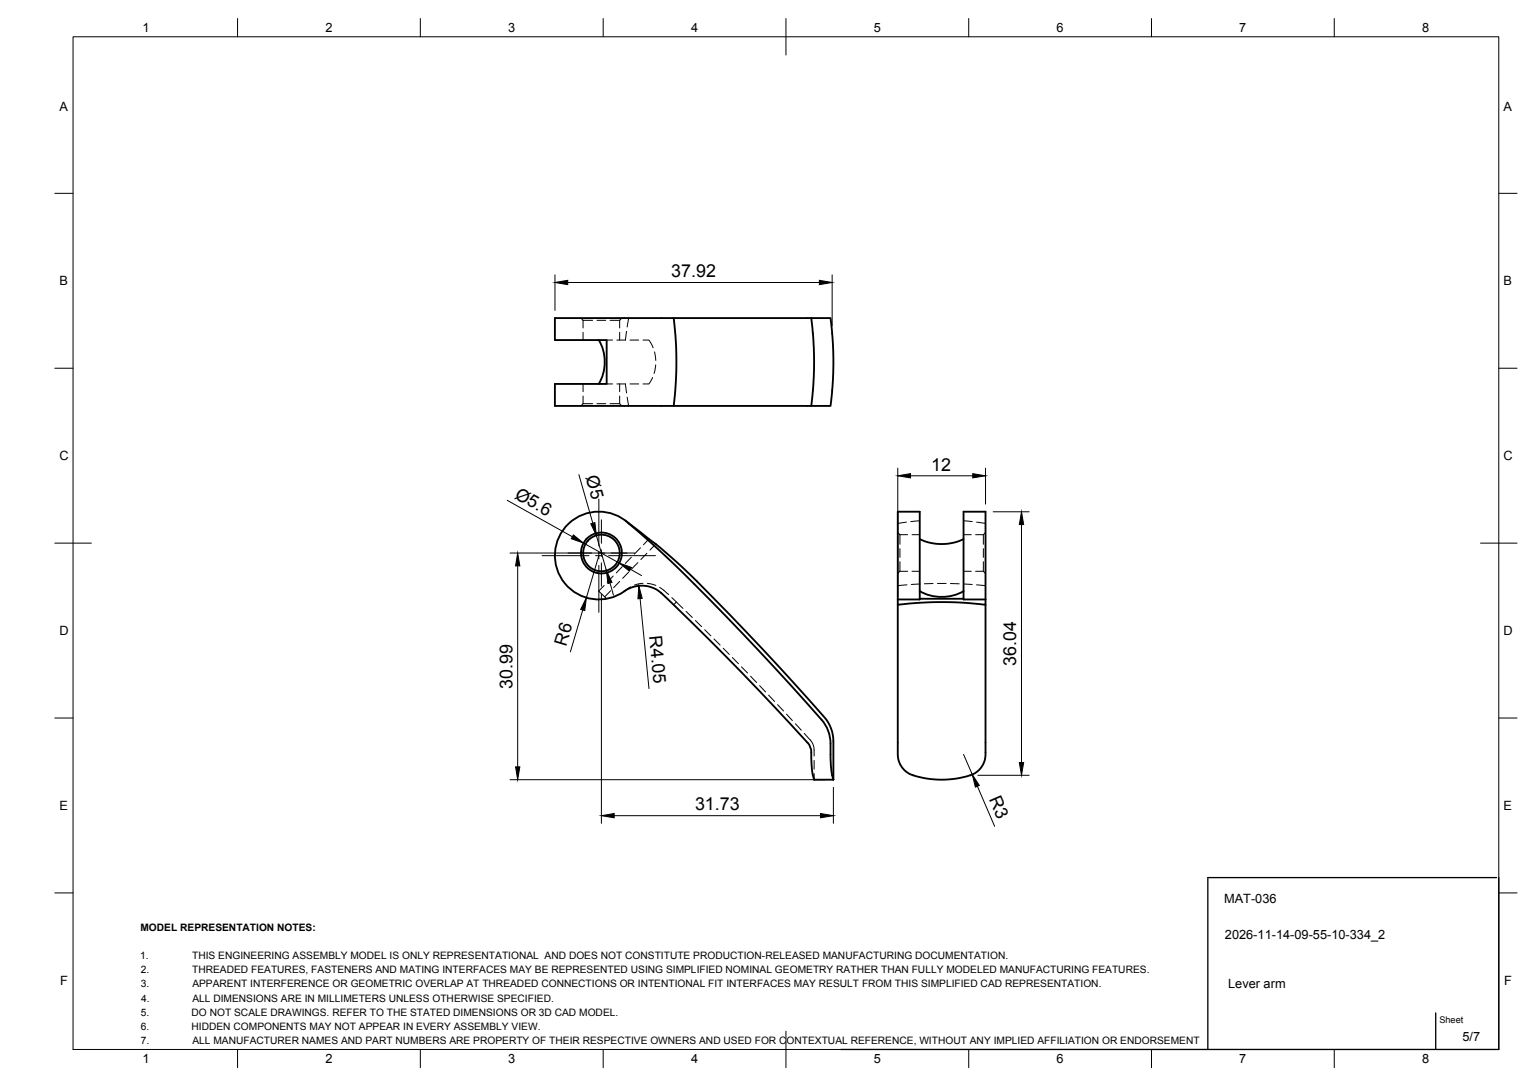
ISO-10303-21;
HEADER;
/* Generated by software containing ST-Developer
 * from STEP Tools, Inc. (www.steptools.com) 
 */

FILE_DESCRIPTION(
/* description */ (''),
/* implementation_level */ '2;1');

FILE_NAME(
/* name */ 'Lever arm.step',
/* time_stamp */ '2026-11-14T09:55:16-08:00',
/* author */ (''),
/* organization */ (''),
/* preprocessor_version */ 'ST-DEVELOPER v20.2',
/* originating_system */ 'Autodesk Translation Framework v15.17.0.0',
/* authorisation */ '');

FILE_SCHEMA (('AUTOMOTIVE_DESIGN { 1 0 10303 214 3 1 1 }'));
ENDSEC;

DATA;
#10=MECHANICAL_DESIGN_GEOMETRIC_PRESENTATION_REPRESENTATION('',(#60),#170250);
#36=B_SPLINE_SURFACE_WITH_KNOTS('',3,3,((#168992,#168993,#168994,#168995),
(#168996,#168997,#168998,#168999),(#169000,#169001,#169002,#169003),(#169004,
#169005,#169006,#169007),(#169008,#169009,#169010,#169011),(#169012,#169013,
#169014,#169015),(#169016,#169017,#169018,#169019),(#169020,#169021,#169022,
#169023),(#169024,#169025,#169026,#169027),(#169028,#169029,#169030,#169031)),
 .UNSPECIFIED.,.F.,.F.,.F.,(4,1,1,1,3,4),(4,4),(0.135790601649557,0.226849968153009,
0.317909334656459,0.40896870115991,0.500028067663362,0.5036704423235),(0.807901539596212,
1.),.UNSPECIFIED.);
#37=B_SPLINE_SURFACE_WITH_KNOTS('',3,3,((#169171,#169172,#169173,#169174,
#169175,#169176,#169177),(#169178,#169179,#169180,#169181,#169182,#169183,
#169184),(#169185,#169186,#169187,#169188,#169189,#169190,#169191),(#169192,
#169193,#169194,#169195,#169196,#169197,#169198),(#169199,#169200,#169201,
#169202,#169203,#169204,#169205),(#169206,#169207,#169208,#169209,#169210,
#169211,#169212),(#169213,#169214,#169215,#169216,#169217,#169218,#169219),
(#169220,#169221,#169222,#169223,#169224,#169225,#169226),(#169227,#169228,
#169229,#169230,#169231,#169232,#169233),(#169234,#169235,#169236,#169237,
#169238,#169239,#169240),(#169241,#169242,#169243,#169244,#169245,#169246,
#169247),(#169248,#169249,#169250,#169251,#169252,#169253,#169254),(#169255,
#169256,#169257,#169258,#169259,#169260,#169261)),.UNSPECIFIED.,.F.,.F.,
 .F.,(4,3,1,1,1,3,4),(4,3,4),(0.114681185572966,0.118496689180301,0.213879533801066,
0.309262378421832,0.404645223042596,0.500028067663362,0.500047049913778),
(-2.58598232202791E-10,0.97179933976621,0.977592668595424),
 .UNSPECIFIED.);
#38=B_SPLINE_SURFACE_WITH_KNOTS('',3,3,((#169612,#169613,#169614,#169615,
#169616,#169617),(#169618,#169619,#169620,#169621,#169622,#169623),(#169624,
#169625,#169626,#169627,#169628,#169629),(#169630,#169631,#169632,#169633,
#169634,#169635),(#169636,#169637,#169638,#169639,#169640,#169641),(#169642,
#169643,#169644,#169645,#169646,#169647),(#169648,#169649,#169650,#169651,
#169652,#169653),(#169654,#169655,#169656,#169657,#169658,#169659),(#169660,
#169661,#169662,#169663,#169664,#169665),(#169666,#169667,#169668,#169669,
#169670,#169671),(#169672,#169673,#169674,#169675,#169676,#169677),(#169678,
#169679,#169680,#169681,#169682,#169683)),.UNSPECIFIED.,.F.,.F.,.F.,(4,
1,1,1,2,1,1,1,4),(4,2,4),(0.618524756843663,0.666209162238205,0.713893567632747,
0.761577973027289,0.809262378421831,0.856946783816374,0.904631189210916,
0.952315594605458,1.),(0.,0.931730586032522,0.937129966266598),
 .UNSPECIFIED.);
#39=B_SPLINE_SURFACE_WITH_KNOTS('',3,3,((#169891,#169892,#169893,#169894),
(#169895,#169896,#169897,#169898),(#169899,#169900,#169901,#169902),(#169903,
#169904,#169905,#169906),(#169907,#169908,#169909,#169910),(#169911,#169912,
#169913,#169914),(#169915,#169916,#169917,#169918),(#169919,#169920,#169921,
#169922),(#169923,#169924,#169925,#169926),(#169927,#169928,#169929,#169930),
(#169931,#169932,#169933,#169934),(#169935,#169936,#169937,#169938),(#169939,
#169940,#169941,#169942),(#169943,#169944,#169945,#169946),(#169947,#169948,
#169949,#169950)),.UNSPECIFIED.,.F.,.F.,.F.,(4,3,1,1,1,2,1,1,1,4),(4,4),
(0.632176856006048,0.635818669312919,0.681341335648804,0.726864001984689,
0.772386668320574,0.81790933465646,0.863432000992345,0.90895466732823,0.954477333664115,
1.),(0.0153819466590792,1.),.UNSPECIFIED.);
#46=SHAPE_REPRESENTATION_RELATIONSHIP('SRR','None',#170278,#52);
#52=ADVANCED_BREP_SHAPE_REPRESENTATION('',(#66),#170246);
#60=STYLED_ITEM('',(#170316),#66);
#66=MANIFOLD_SOLID_BREP('Body1',#71400);
#76=FACE_BOUND('',#15893,.T.);
#77=FACE_BOUND('',#15895,.T.);
#78=FACE_BOUND('',#15897,.T.);
#79=FACE_BOUND('',#15901,.T.);
#98=PLANE('',#77702);
#99=PLANE('',#77704);
#100=PLANE('',#77706);
#101=PLANE('',#77707);
#102=PLANE('',#77710);
#192=ELLIPSE('',#77705,65.55169862647,42.389902647677);
#193=ELLIPSE('',#77708,65.5506952259048,42.388915448489);
#4370=(
BOUNDED_SURFACE()
B_SPLINE_SURFACE(3,1,((#168511,#168512),(#168513,#168514),(#168515,#168516),
(#168517,#168518)),.UNSPECIFIED.,.F.,.F.,.F.)
B_SPLINE_SURFACE_WITH_KNOTS((4,4),(2,2),(-8.56707287333166E-8,1.00000008548767),
(0.00592879452423504,0.99406998347921),.UNSPECIFIED.)
GEOMETRIC_REPRESENTATION_ITEM()
RATIONAL_B_SPLINE_SURFACE(((1.00000000253644,1.00000000253644),(0.990131033425531,
0.990131033425531),(0.990131033423724,0.990131033423724),(1.00000000253103,
1.00000000253102)))
REPRESENTATION_ITEM('')
SURFACE()
);
#4371=(
BOUNDED_SURFACE()
B_SPLINE_SURFACE(3,2,((#168680,#168681,#168682),(#168683,#168684,#168685),
(#168686,#168687,#168688),(#168689,#168690,#168691),(#168692,#168693,#168694),
(#168695,#168696,#168697),(#168698,#168699,#168700),(#168701,#168702,#168703),
(#168704,#168705,#168706),(#168707,#168708,#168709),(#168710,#168711,#168712),
(#168713,#168714,#168715),(#168716,#168717,#168718),(#168719,#168720,#168721),
(#168722,#168723,#168724),(#168725,#168726,#168727),(#168728,#168729,#168730),
(#168731,#168732,#168733),(#168734,#168735,#168736),(#168737,#168738,#168739),
(#168740,#168741,#168742),(#168743,#168744,#168745),(#168746,#168747,#168748),
(#168749,#168750,#168751),(#168752,#168753,#168754),(#168755,#168756,#168757),
(#168758,#168759,#168760),(#168761,#168762,#168763),(#168764,#168765,#168766),
(#168767,#168768,#168769),(#168770,#168771,#168772),(#168773,#168774,#168775),
(#168776,#168777,#168778),(#168779,#168780,#168781),(#168782,#168783,#168784),
(#168785,#168786,#168787),(#168788,#168789,#168790),(#168791,#168792,#168793),
(#168794,#168795,#168796),(#168797,#168798,#168799),(#168800,#168801,#168802),
(#168803,#168804,#168805),(#168806,#168807,#168808),(#168809,#168810,#168811),
(#168812,#168813,#168814),(#168815,#168816,#168817),(#168818,#168819,#168820),
(#168821,#168822,#168823),(#168824,#168825,#168826),(#168827,#168828,#168829)),
 .UNSPECIFIED.,.F.,.F.,.F.)
B_SPLINE_SURFACE_WITH_KNOTS((4,2,2,2,2,2,2,2,2,2,2,2,2,2,2,2,2,2,2,2,2,
2,2,2,4),(3,3),(0.00438204809785496,0.00442773757395586,0.00445058231200631,
0.00446200468103154,0.00447342705005676,0.00451911652615766,0.00454196126420811,
0.00456480600225856,0.00474756390666215,0.00511307971546933,0.0058441113330837,
0.00730617456831243,0.0102303010387699,0.0131544275092274,0.0146164907444561,
0.0153475223620705,0.0157130381708776,0.0158957960752812,0.0159186408133317,
0.0159414855513821,0.015987175027483,0.0159985973965083,0.0160100197655335,
0.0160328645035839,0.0160785539796848),(0.,1.),.UNSPECIFIED.)
GEOMETRIC_REPRESENTATION_ITEM()
RATIONAL_B_SPLINE_SURFACE(((1.,0.934218767962417,1.),(1.,0.934219268725543,
1.),(1.,0.934219769475696,1.),(1.,0.934220520581468,1.),(1.,0.934221098516136,
1.),(1.,0.93422098270531,1.),(1.,0.934218146084782,1.),(1.,0.934214890227589,
1.),(1.,0.934213259806577,1.),(1.,0.934205095242336,1.),(1.,0.934198523721367,
1.),(1.,0.934188606688787,1.),(1.,0.934185286091514,1.),(1.,0.934178648365384,
1.),(1.,0.934175336166584,1.),(1.,0.934145586350039,1.),(1.,0.934119568538277,
1.),(1.,0.934042793646304,1.),(1.,0.933993312945644,1.),(1.,0.933849992791617,
1.),(1.,0.933761355730532,1.),(1.,0.93351603018512,1.),(1.,0.933379914807182,
1.),(1.,0.93305317905279,1.),(1.,0.932943966614937,1.),(1.,0.932943963043387,
1.),(1.,0.933053175643618,1.),(1.,0.933379911515294,1.),(1.,0.93351602735766,
1.),(1.,0.933761354538682,1.),(1.,0.933849992301547,1.),(1.,0.933993313783528,
1.),(1.,0.93404279394322,1.),(1.,0.934119568707732,1.),(1.,0.934145586476303,
1.),(1.,0.934175336243606,1.),(1.,0.934178648436936,1.),(1.,0.934185286152106,
1.),(1.,0.934188606743602,1.),(1.,0.934198523759289,1.),(1.,0.9342050952691,
1.),(1.,0.934213259819631,1.),(1.,0.934214890237893,1.),(1.,0.934218146089636,
1.),(1.,0.934220982704232,1.),(1.,0.934221098518431,1.),(1.,0.934220520582345,
1.),(1.,0.934219769477844,1.),(1.,0.934219268728507,1.),(1.,0.934218767966226,
1.)))
REPRESENTATION_ITEM('')
SURFACE()
);
#4372=(
BOUNDED_SURFACE()
B_SPLINE_SURFACE(3,1,((#168914,#168915),(#168916,#168917),(#168918,#168919),
(#168920,#168921)),.UNSPECIFIED.,.F.,.F.,.F.)
B_SPLINE_SURFACE_WITH_KNOTS((4,4),(2,2),(-8.59560614834357E-8,1.00000008613876),
(0.00592875831867496,0.994072405691805),.UNSPECIFIED.)
GEOMETRIC_REPRESENTATION_ITEM()
RATIONAL_B_SPLINE_SURFACE(((1.00000000254489,1.00000000254489),(0.990131033419105,
0.990131033419106),(0.990131033420908,0.990131033420909),(1.0000000025503,
1.0000000025503)))
REPRESENTATION_ITEM('')
SURFACE()
);
#4373=(
BOUNDED_SURFACE()
B_SPLINE_SURFACE(3,2,((#169270,#169271,#169272),(#169273,#169274,#169275),
(#169276,#169277,#169278),(#169279,#169280,#169281),(#169282,#169283,#169284),
(#169285,#169286,#169287),(#169288,#169289,#169290),(#169291,#169292,#169293),
(#169294,#169295,#169296),(#169297,#169298,#169299),(#169300,#169301,#169302),
(#169303,#169304,#169305),(#169306,#169307,#169308),(#169309,#169310,#169311),
(#169312,#169313,#169314),(#169315,#169316,#169317),(#169318,#169319,#169320),
(#169321,#169322,#169323),(#169324,#169325,#169326),(#169327,#169328,#169329),
(#169330,#169331,#169332),(#169333,#169334,#169335),(#169336,#169337,#169338),
(#169339,#169340,#169341),(#169342,#169343,#169344),(#169345,#169346,#169347),
(#169348,#169349,#169350),(#169351,#169352,#169353),(#169354,#169355,#169356),
(#169357,#169358,#169359),(#169360,#169361,#169362),(#169363,#169364,#169365),
(#169366,#169367,#169368),(#169369,#169370,#169371),(#169372,#169373,#169374),
(#169375,#169376,#169377),(#169378,#169379,#169380),(#169381,#169382,#169383),
(#169384,#169385,#169386),(#169387,#169388,#169389),(#169390,#169391,#169392),
(#169393,#169394,#169395),(#169396,#169397,#169398),(#169399,#169400,#169401),
(#169402,#169403,#169404),(#169405,#169406,#169407),(#169408,#169409,#169410),
(#169411,#169412,#169413),(#169414,#169415,#169416),(#169417,#169418,#169419),
(#169420,#169421,#169422),(#169423,#169424,#169425),(#169426,#169427,#169428),
(#169429,#169430,#169431),(#169432,#169433,#169434),(#169435,#169436,#169437),
(#169438,#169439,#169440),(#169441,#169442,#169443),(#169444,#169445,#169446),
(#169447,#169448,#169449),(#169450,#169451,#169452),(#169453,#169454,#169455),
(#169456,#169457,#169458),(#169459,#169460,#169461),(#169462,#169463,#169464),
(#169465,#169466,#169467),(#169468,#169469,#169470),(#169471,#169472,#169473),
(#169474,#169475,#169476),(#169477,#169478,#169479),(#169480,#169481,#169482),
(#169483,#169484,#169485),(#169486,#169487,#169488),(#169489,#169490,#169491)),
 .UNSPECIFIED.,.F.,.F.,.F.)
B_SPLINE_SURFACE_WITH_KNOTS((4,2,2,2,2,2,2,2,2,2,2,2,2,2,2,2,2,2,2,2,2,
2,2,2,2,2,2,2,2,2,2,2,2,2,2,2,4),(3,3),(0.0179612750605611,0.0180038120055911,
0.0180250804781061,0.0180303975962348,0.0180357147143635,0.018046348950621,
0.0181314228406809,0.0182164967307408,0.0182271309669983,0.0182377652032558,
0.0182590336757708,0.0183015706208007,0.0186418661810403,0.0193224573015194,
0.0200030484219985,0.0206836395424776,0.0213642306629567,0.0220448217834359,
0.0234060040243941,0.0247671862653523,0.0254477773858315,0.0261283685063106,
0.0268089596267897,0.0274895507472688,0.0281701418677479,0.0285104374279875,
0.0285529743730174,0.0285742428455324,0.0285848770817899,0.0285955113180474,
0.0286805852081073,0.0287656590981672,0.0287762933344247,0.0287816104525534,
0.0287869275706821,0.0288081960431971,0.0288507329882271),(0.,1.),
 .UNSPECIFIED.)
GEOMETRIC_REPRESENTATION_ITEM()
RATIONAL_B_SPLINE_SURFACE(((1.,0.936904821453696,1.),(1.,0.936904794108661,
1.),(1.,0.936904766764048,1.),(1.,0.936904725747745,1.),(1.,0.936905128260374,
1.),(1.,0.936904590939729,1.),(1.,0.936903346459592,1.),(1.,0.936901627765994,
1.),(1.,0.936900767797278,1.),(1.,0.936898186025644,1.),(1.,0.936896462357224,
1.),(1.,0.936880926961442,1.),(1.,0.936866958574279,1.),(1.,0.936838704163249,
1.),(1.,0.936824418139244,1.),(1.,0.936808168049907,1.),(1.,0.936806360007847,
1.),(1.,0.936802738971814,1.),(1.,0.936800862095946,1.),(1.,0.936795849431034,
1.),(1.,0.936792514575336,1.),(1.,0.936782530740213,1.),(1.,0.936775902492467,
1.),(1.,0.936716496356665,1.),(1.,0.936665452813206,1.),(1.,0.936517538966925,
1.),(1.,0.93642586040289,1.),(1.,0.936256634386565,1.),(1.,0.936179189842934,
1.),(1.,0.936038226722045,1.),(1.,0.935974776717855,1.),(1.,0.935862123528188,
1.),(1.,0.935812981619732,1.),(1.,0.93572859095576,1.),(1.,0.935693341074582,
1.),(1.,0.935608906032864,1.),(1.,0.935580787501173,1.),(1.,0.935580755598083,
1.),(1.,0.935608926183175,1.),(1.,0.935693493416876,1.),(1.,0.935728787043659,
1.),(1.,0.935813225027166,1.),(1.,0.935862370889367,1.),(1.,0.935974951078453,
1.),(1.,0.936038323852223,1.),(1.,0.936179015169328,1.),(1.,0.93625634937854,
1.),(1.,0.936425491452454,1.),(1.,0.936517220625567,1.),(1.,0.936665263045723,
1.),(1.,0.9367163495052,1.),(1.,0.936775803162665,1.),(1.,0.936782436680194,
1.),(1.,0.936792428402367,1.),(1.,0.936795765884152,1.),(1.,0.936800782483542,
1.),(1.,0.936802654166495,1.),(1.,0.936806278312161,1.),(1.,0.936808087904325,
1.),(1.,0.936824351902175,1.),(1.,0.936838649987733,1.),(1.,0.936866927922814,
1.),(1.,0.936880907772467,1.),(1.,0.93689645572885,1.),(1.,0.936898180788246,
1.),(1.,0.936900764639372,1.),(1.,0.936901625300091,1.),(1.,0.936903345375374,
1.),(1.,0.936904591114425,1.),(1.,0.936905127567446,1.),(1.,0.936904725770864,
1.),(1.,0.936904766820085,1.),(1.,0.93690479418665,1.),(1.,0.936904821553629,
1.)))
REPRESENTATION_ITEM('')
SURFACE()
);
#4374=(
BOUNDED_SURFACE()
B_SPLINE_SURFACE(3,2,((#169695,#169696,#169697),(#169698,#169699,#169700),
(#169701,#169702,#169703),(#169704,#169705,#169706),(#169707,#169708,#169709),
(#169710,#169711,#169712),(#169713,#169714,#169715),(#169716,#169717,#169718),
(#169719,#169720,#169721),(#169722,#169723,#169724),(#169725,#169726,#169727),
(#169728,#169729,#169730),(#169731,#169732,#169733),(#169734,#169735,#169736),
(#169737,#169738,#169739),(#169740,#169741,#169742),(#169743,#169744,#169745),
(#169746,#169747,#169748),(#169749,#169750,#169751),(#169752,#169753,#169754),
(#169755,#169756,#169757),(#169758,#169759,#169760),(#169761,#169762,#169763),
(#169764,#169765,#169766),(#169767,#169768,#169769),(#169770,#169771,#169772),
(#169773,#169774,#169775),(#169776,#169777,#169778),(#169779,#169780,#169781),
(#169782,#169783,#169784),(#169785,#169786,#169787),(#169788,#169789,#169790),
(#169791,#169792,#169793),(#169794,#169795,#169796),(#169797,#169798,#169799),
(#169800,#169801,#169802),(#169803,#169804,#169805),(#169806,#169807,#169808),
(#169809,#169810,#169811),(#169812,#169813,#169814),(#169815,#169816,#169817),
(#169818,#169819,#169820),(#169821,#169822,#169823),(#169824,#169825,#169826),
(#169827,#169828,#169829),(#169830,#169831,#169832),(#169833,#169834,#169835),
(#169836,#169837,#169838),(#169839,#169840,#169841),(#169842,#169843,#169844),
(#169845,#169846,#169847),(#169848,#169849,#169850)),.UNSPECIFIED.,.F.,
 .F.,.F.)
B_SPLINE_SURFACE_WITH_KNOTS((4,2,2,2,2,2,2,2,2,2,2,2,2,2,2,2,2,2,2,2,2,
2,2,2,2,4),(3,3),(0.0156015153159842,0.0159832133339201,0.0161740623428881,
0.016269486847372,0.016317199099614,0.016341055225735,0.0163529832887955,
0.016364911351856,0.0171283073877279,0.0186550994594716,0.0194184954953434,
0.0201818915312153,0.021708683602959,0.0224720796388308,0.0232354756747027,
0.0247622677464464,0.0262890598181901,0.0270524558540619,0.0270584198855922,
0.0270643839171224,0.0270763119801829,0.0271001681063039,0.0271478803585459,
0.0272433048630299,0.0274341538719979,0.0278158518899338),(0.,1.),
 .UNSPECIFIED.)
GEOMETRIC_REPRESENTATION_ITEM()
RATIONAL_B_SPLINE_SURFACE(((1.,0.776444097652961,1.),(1.,0.776058926606058,
1.),(1.,0.775673843099958,1.),(1.,0.775096481210286,1.),(1.,0.774904071156476,
1.),(1.,0.774615538680226,1.),(1.,0.774519374957158,1.),(1.,0.774375152135543,
1.),(1.,0.774327081655569,1.),(1.,0.774254981891155,1.),(1.,0.774230949628936,
1.),(1.,0.774194902757698,1.),(1.,0.774182887387605,1.),(1.,0.774158857160334,
1.),(1.,0.774150992177244,1.),(1.,0.773543654478887,1.),(1.,0.77298505575604,
1.),(1.,0.771431978714256,1.),(1.,0.77056039765908,1.),(1.,0.769511352915782,
1.),(1.,0.769204886519117,1.),(1.,0.768679727581747,1.),(1.,0.768460849050857,
1.),(1.,0.767935355999606,1.),(1.,0.767759786976898,1.),(1.,0.767759465570472,
1.),(1.,0.767803217713065,1.),(1.,0.767978602526777,1.),(1.,0.768110252004706,
1.),(1.,0.768636034778269,1.),(1.,0.769161202927011,1.),(1.,0.770557236848331,
1.),(1.,0.771427908462379,1.),(1.,0.772982352753207,1.),(1.,0.773541690771539,
1.),(1.,0.774144848886315,1.),(1.,0.774149526925736,1.),(1.,0.774158887792997,
1.),(1.,0.77416299521755,1.),(1.,0.774181034357718,1.),(1.,0.774193060706593,
1.),(1.,0.774229140511077,1.),(1.,0.774253194724663,1.),(1.,0.774325360330513,
1.),(1.,0.774373474688076,1.),(1.,0.774517829090711,1.),(1.,0.774614080465712,
1.),(1.,0.774902875681382,1.),(1.,0.775095460606343,1.),(1.,0.775673346165181,
1.),(1.,0.776058777525586,1.),(1.,0.776444294966368,1.)))
REPRESENTATION_ITEM('')
SURFACE()
);
#4458=(
BOUNDED_CURVE()
B_SPLINE_CURVE(3,(#168924,#168925,#168926,#168927,#168928,#168929,#168930,
#168931,#168932,#168933,#168934,#168935,#168936,#168937,#168938,#168939,
#168940,#168941,#168942,#168943,#168944,#168945,#168946,#168947,#168948,
#168949,#168950,#168951,#168952,#168953,#168954,#168955,#168956,#168957,
#168958,#168959,#168960,#168961,#168962,#168963,#168964,#168965,#168966,
#168967,#168968,#168969,#168970,#168971,#168972,#168973,#168974,#168975,
#168976,#168977,#168978,#168979,#168980,#168981,#168982,#168983,#168984,
#168985,#168986,#168987,#168988,#168989),.UNSPECIFIED.,.F.,.F.)
B_SPLINE_CURVE_WITH_KNOTS((4,2,2,2,2,2,2,2,2,2,2,2,2,2,2,2,2,2,2,2,2,2,
2,2,2,2,2,2,2,2,2,2,4),(0.,0.000426248299516627,0.000920386532912638,0.00190866299971401,
0.00981487473411692,0.0177210864685195,0.0187093629353212,0.0196976394021223,
0.0216741923357257,0.0256272982029221,0.0572521451405331,0.120501839015745,
0.183751532890957,0.24700122676617,0.310250920641382,0.373500614516604,
0.500000002267029,0.626499390017453,0.689749083892675,0.752998777767887,
0.816248471643099,0.879498165518312,0.942747859393524,0.974372706331135,
0.978325812198331,0.980302365131934,0.981290641598736,0.982278918065537,
0.99018512979994,0.998091341534343,0.999079618001144,0.99957375623454,1.),
 .UNSPECIFIED.)
CURVE()
GEOMETRIC_REPRESENTATION_ITEM()
RATIONAL_B_SPLINE_CURVE((0.999999893495044,0.999999893494474,0.999999893492739,
0.999999893490038,0.999999893488586,0.999999893484228,0.999999893481318,
0.999999893455095,0.999999893431516,0.999999893383822,0.999999893359708,
0.999999893332278,0.999999893329226,0.999999893323113,0.999999893319945,
0.999999893311484,0.999999893305855,0.999999893289002,0.999999893277814,
0.999999893177536,0.999999893091374,0.999999892841696,0.999999892686943,
0.99999989240129,0.999999892270563,0.999999892032618,0.999999891925514,
0.999999891735356,0.999999891652404,0.999999891509953,0.999999891450451,
0.999999891307925,0.999999891260461,0.999999891260407,0.999999891307959,
0.999999891450708,0.999999891510284,0.999999891652815,0.999999891735774,
0.999999891925809,0.999999892032782,0.999999892270268,0.999999892400809,
0.99999989268632,0.999999892841159,0.999999893091054,0.999999893177288,
0.999999893277646,0.999999893288843,0.999999893305709,0.999999893311343,
0.999999893319811,0.99999989332297,0.999999893329088,0.999999893332142,
0.999999893359596,0.999999893383731,0.999999893431464,0.999999893455062,
0.999999893481307,0.999999893484219,0.99999989348858,0.999999893490033,
0.999999893492737,0.999999893494474,0.999999893495044))
REPRESENTATION_ITEM('')
);
#5369=CYLINDRICAL_SURFACE('',#77682,2.5);
#5370=CYLINDRICAL_SURFACE('',#77689,2.5);
#5371=CYLINDRICAL_SURFACE('',#77691,12.9999999996215);
#5372=CYLINDRICAL_SURFACE('',#77694,6.00000000044796);
#5373=CYLINDRICAL_SURFACE('',#77699,2.99999999919632);
#5374=CYLINDRICAL_SURFACE('',#77700,2.99999999919632);
#5375=CYLINDRICAL_SURFACE('',#77709,4.50000000012307);
#10604=FACE_OUTER_BOUND('',#15875,.T.);
#10605=FACE_OUTER_BOUND('',#15876,.T.);
#10606=FACE_OUTER_BOUND('',#15877,.T.);
#10607=FACE_OUTER_BOUND('',#15878,.T.);
#10608=FACE_OUTER_BOUND('',#15879,.T.);
#10609=FACE_OUTER_BOUND('',#15880,.T.);
#10610=FACE_OUTER_BOUND('',#15881,.T.);
#10611=FACE_OUTER_BOUND('',#15882,.T.);
#10612=FACE_OUTER_BOUND('',#15883,.T.);
#10613=FACE_OUTER_BOUND('',#15884,.T.);
#10614=FACE_OUTER_BOUND('',#15885,.T.);
#10615=FACE_OUTER_BOUND('',#15886,.T.);
#10616=FACE_OUTER_BOUND('',#15887,.T.);
#10617=FACE_OUTER_BOUND('',#15888,.T.);
#10618=FACE_OUTER_BOUND('',#15889,.T.);
#10619=FACE_OUTER_BOUND('',#15890,.T.);
#10620=FACE_OUTER_BOUND('',#15891,.T.);
#10621=FACE_OUTER_BOUND('',#15892,.T.);
#10622=FACE_OUTER_BOUND('',#15894,.T.);
#10623=FACE_OUTER_BOUND('',#15896,.T.);
#10624=FACE_OUTER_BOUND('',#15898,.T.);
#10625=FACE_OUTER_BOUND('',#15899,.T.);
#10626=FACE_OUTER_BOUND('',#15900,.T.);
#15875=EDGE_LOOP('',(#65778,#65779,#65780,#65781,#65782));
#15876=EDGE_LOOP('',(#65783,#65784,#65785,#65786));
#15877=EDGE_LOOP('',(#65787,#65788,#65789,#65790));
#15878=EDGE_LOOP('',(#65791,#65792,#65793,#65794));
#15879=EDGE_LOOP('',(#65795,#65796,#65797,#65798,#65799));
#15880=EDGE_LOOP('',(#65800,#65801,#65802,#65803,#65804,#65805,#65806,#65807));
#15881=EDGE_LOOP('',(#65808,#65809,#65810,#65811,#65812,#65813));
#15882=EDGE_LOOP('',(#65814,#65815,#65816,#65817));
#15883=EDGE_LOOP('',(#65818,#65819,#65820,#65821));
#15884=EDGE_LOOP('',(#65822,#65823,#65824,#65825));
#15885=EDGE_LOOP('',(#65826,#65827,#65828,#65829,#65830,#65831));
#15886=EDGE_LOOP('',(#65832,#65833,#65834,#65835));
#15887=EDGE_LOOP('',(#65836,#65837,#65838,#65839));
#15888=EDGE_LOOP('',(#65840,#65841,#65842,#65843));
#15889=EDGE_LOOP('',(#65844,#65845,#65846,#65847));
#15890=EDGE_LOOP('',(#65848,#65849,#65850,#65851));
#15891=EDGE_LOOP('',(#65852,#65853,#65854,#65855));
#15892=EDGE_LOOP('',(#65856,#65857,#65858,#65859));
#15893=EDGE_LOOP('',(#65860));
#15894=EDGE_LOOP('',(#65861,#65862,#65863,#65864,#65865,#65866,#65867,#65868,
#65869,#65870,#65871));
#15895=EDGE_LOOP('',(#65872));
#15896=EDGE_LOOP('',(#65873,#65874,#65875,#65876,#65877,#65878,#65879,#65880,
#65881,#65882,#65883));
#15897=EDGE_LOOP('',(#65884));
#15898=EDGE_LOOP('',(#65885,#65886,#65887,#65888,#65889,#65890,#65891,#65892));
#15899=EDGE_LOOP('',(#65893,#65894,#65895,#65896));
#15900=EDGE_LOOP('',(#65897,#65898,#65899,#65900));
#15901=EDGE_LOOP('',(#65901));
#21011=CIRCLE('',#77683,2.5);
#21012=CIRCLE('',#77684,2.5);
#21013=CIRCLE('',#77685,2.5);
#21014=CIRCLE('',#77687,2.50000000008162);
#21015=CIRCLE('',#77688,2.79999999966249);
#21016=CIRCLE('',#77690,2.5);
#21017=CIRCLE('',#77693,2.79999999971483);
#21018=CIRCLE('',#77695,6.00000000044796);
#21019=CIRCLE('',#77696,6.00000000044796);
#21020=CIRCLE('',#77697,6.00000000044794);
#21021=CIRCLE('',#77698,6.00000000044795);
#21022=CIRCLE('',#77701,35.000000093214);
#21023=CIRCLE('',#77703,4.50000000012307);
#24318=B_SPLINE_CURVE_WITH_KNOTS('',3,(#168405,#168406,#168407,#168408,
#168409,#168410,#168411,#168412,#168413,#168414),.UNSPECIFIED.,.F.,.F.,
(4,2,2,2,4),(9.99999999599415E-7,0.199896964270254,0.396819956928882,0.593738515946119,
0.793630665235622),.UNSPECIFIED.);
#24319=B_SPLINE_CURVE_WITH_KNOTS('',3,(#168418,#168419,#168420,#168421,
#168422,#168423,#168424,#168425,#168426,#168427),.UNSPECIFIED.,.F.,.F.,
(4,2,2,2,4),(1.0000000102557E-6,0.212494298875736,0.396821009247289,0.581148812864389,
0.793634316910742),.UNSPECIFIED.);
#24320=B_SPLINE_CURVE_WITH_KNOTS('',3,(#168438,#168439,#168440,#168441,
#168442,#168443),.UNSPECIFIED.,.F.,.F.,(4,2,4),(3.14399518292747E-10,0.174984677416615,
0.304359067388048),.UNSPECIFIED.);
#24321=B_SPLINE_CURVE_WITH_KNOTS('',3,(#168451,#168452,#168453,#168454,
#168455,#168456),.UNSPECIFIED.,.F.,.F.,(4,2,4),(0.000105555394099198,0.130107181442079,
0.280405013941638),.UNSPECIFIED.);
#24322=B_SPLINE_CURVE_WITH_KNOTS('',3,(#168459,#168460,#168461,#168462,
#168463,#168464,#168465,#168466,#168467,#168468,#168469,#168470,#168471,
#168472,#168473,#168474,#168475,#168476,#168477,#168478,#168479,#168480,
#168481,#168482,#168483,#168484,#168485,#168486,#168487,#168488,#168489,
#168490,#168491,#168492,#168493,#168494,#168495,#168496,#168497,#168498,
#168499,#168500,#168501,#168502,#168503,#168504,#168505,#168506,#168507,
#168508,#168509,#168510),.UNSPECIFIED.,.F.,.F.,(4,2,2,2,2,2,2,2,2,2,2,2,
2,2,2,2,2,2,2,2,2,2,2,2,2,4),(0.,0.0256250094143976,0.0414375088162371,
0.0493437585171568,0.053296883367617,0.0552734457928468,0.0562617270054617,
0.056755867611765,0.0572500082180766,0.120500005825418,0.247000001040109,
0.373499996254801,0.43674999386215,0.499999991469491,0.626499986684183,
0.689749984291532,0.752999981898873,0.879499977113565,0.942749974720914,
0.943738255933529,0.944726537146144,0.946703099571374,0.950656224421834,
0.958562474122746,0.974374973524585,0.999999995455179),.UNSPECIFIED.);
#24323=B_SPLINE_CURVE_WITH_KNOTS('',3,(#168520,#168521,#168522,#168523,
#168524,#168525,#168526,#168527,#168528,#168529),.UNSPECIFIED.,.F.,.F.,
(4,2,2,2,4),(-0.381457606174089,-0.304035109378442,-0.190979808271481,-0.0912225470703838,
-1.00000006925116E-6),.UNSPECIFIED.);
#24324=B_SPLINE_CURVE_WITH_KNOTS('',3,(#168533,#168534,#168535,#168536,
#168537,#168538,#168539,#168540,#168541,#168542,#168543,#168544,#168545,
#168546,#168547,#168548,#168549,#168550,#168551,#168552,#168553,#168554,
#168555,#168556,#168557,#168558,#168559,#168560,#168561,#168562,#168563,
#168564,#168565,#168566,#168567,#168568,#168569,#168570,#168571,#168572,
#168573,#168574,#168575,#168576,#168577,#168578,#168579,#168580,#168581,
#168582,#168583,#168584,#168585,#168586,#168587,#168588,#168589,#168590,
#168591,#168592,#168593,#168594,#168595,#168596,#168597,#168598,#168599,
#168600,#168601,#168602,#168603,#168604,#168605,#168606,#168607,#168608,
#168609,#168610,#168611,#168612,#168613,#168614,#168615,#168616,#168617,
#168618,#168619,#168620,#168621,#168622,#168623,#168624,#168625,#168626,
#168627,#168628,#168629,#168630,#168631,#168632,#168633,#168634,#168635,
#168636,#168637,#168638,#168639,#168640,#168641),.UNSPECIFIED.,.F.,.F.,
(4,3,3,3,3,3,3,3,3,3,3,3,3,3,3,3,3,3,3,3,3,3,3,3,3,3,3,3,3,3,3,3,3,3,3,
3,4),(0.,0.000877428960298162,0.00182186904808312,0.00560425316389786,0.00749819548399555,
0.00939395278983934,0.0246236265420485,0.0553976406888011,0.10510590613333,
0.117953721761098,0.16822163443711,0.218581997077039,0.244710640454446,
0.25,0.350381617416015,0.448693290958287,0.484375,0.498632474707576,0.49999999286025,
0.50105084551746,0.601647811048279,0.624999999999999,0.725405038227879,
0.746093749999999,0.749999999999999,0.753208507973121,0.875,0.883895257725269,
0.918382175878415,0.946288347314178,0.976389806038248,0.991048440539466,
0.99286064175195,0.994668244628355,0.998269520917499,0.999166914580596,
0.999999987137999),.UNSPECIFIED.);
#24325=B_SPLINE_CURVE_WITH_KNOTS('',3,(#168644,#168645,#168646,#168647,
#168648,#168649,#168650,#168651,#168652,#168653),.UNSPECIFIED.,.F.,.F.,
(4,2,2,2,4),(-0.381485937812174,-0.290460031477783,-0.190961318136168,-0.0775891327103021,
-1.00000005109901E-6),.UNSPECIFIED.);
#24326=B_SPLINE_CURVE_WITH_KNOTS('',3,(#168657,#168658,#168659,#168660,
#168661,#168662,#168663,#168664,#168665,#168666),.UNSPECIFIED.,.F.,.F.,
(4,2,2,2,4),(1.00000006872122E-6,0.0915138874962241,0.190511167453547,0.301327535855596,
0.381447321977382),.UNSPECIFIED.);
#24327=B_SPLINE_CURVE_WITH_KNOTS('',3,(#168670,#168671,#168672,#168673,
#168674,#168675,#168676,#168677,#168678,#168679),.UNSPECIFIED.,.F.,.F.,
(4,2,2,2,4),(1.00000005224979E-6,0.0799606858619584,0.19048250138979,0.289749093438666,
0.381474629767968),.UNSPECIFIED.);
#24328=B_SPLINE_CURVE_WITH_KNOTS('',3,(#168832,#168833,#168834,#168835,
#168836,#168837,#168838,#168839,#168840,#168841,#168842,#168843,#168844,
#168845,#168846,#168847,#168848,#168849,#168850,#168851,#168852,#168853,
#168854,#168855,#168856,#168857,#168858,#168859,#168860,#168861,#168862,
#168863,#168864,#168865,#168866,#168867,#168868,#168869,#168870,#168871,
#168872,#168873,#168874,#168875,#168876,#168877,#168878,#168879,#168880,
#168881,#168882,#168883,#168884,#168885,#168886,#168887,#168888,#168889,
#168890,#168891,#168892,#168893,#168894,#168895,#168896,#168897,#168898,
#168899,#168900,#168901),.UNSPECIFIED.,.F.,.F.,(4,3,3,3,3,3,3,3,3,3,3,3,
3,3,3,3,3,3,3,3,3,3,3,4),(0.,0.000547902305461683,0.00249435877321915,0.0180971390547113,
0.0494623915149704,0.112771098950549,0.184521296536466,0.241157246478698,
0.313497254092451,0.385778846725024,0.457780221042424,0.5,0.500001064694345,
0.572039858897225,0.644277278226495,0.716628202259504,0.758843661753893,
0.830600495604986,0.887229062947173,0.950537595516011,0.981902833679206,
0.99750562749206,0.999452086664773,1.),.UNSPECIFIED.);
#24329=B_SPLINE_CURVE_WITH_KNOTS('',3,(#168902,#168903,#168904,#168905,
#168906,#168907),.UNSPECIFIED.,.F.,.F.,(4,2,4),(-0.146653736581323,-0.073340873363055,
-2.14074661886166E-8),.UNSPECIFIED.);
#24330=B_SPLINE_CURVE_WITH_KNOTS('',3,(#168908,#168909,#168910,#168911,
#168912,#168913),.UNSPECIFIED.,.F.,.F.,(4,2,4),(2.14415571569341E-8,0.0733336158677515,
0.146653733111165),.UNSPECIFIED.);
#24331=B_SPLINE_CURVE_WITH_KNOTS('',3,(#169034,#169035,#169036,#169037),
 .UNSPECIFIED.,.F.,.F.,(4,4),(0.,0.00231659945791558),.UNSPECIFIED.);
#24332=B_SPLINE_CURVE_WITH_KNOTS('',3,(#169039,#169040,#169041,#169042,
#169043,#169044),.UNSPECIFIED.,.F.,.F.,(4,2,4),(3.0808796214308E-11,0.603462743313919,
1.20583125094992),.UNSPECIFIED.);
#24333=B_SPLINE_CURVE_WITH_KNOTS('',3,(#169046,#169047,#169048,#169049),
 .UNSPECIFIED.,.F.,.F.,(4,4),(0.,0.00231659459060812),.UNSPECIFIED.);
#24334=B_SPLINE_CURVE_WITH_KNOTS('',3,(#169050,#169051,#169052,#169053,
#169054,#169055,#169056,#169057,#169058,#169059,#169060,#169061,#169062,
#169063,#169064,#169065,#169066,#169067,#169068,#169069,#169070,#169071,
#169072,#169073,#169074,#169075,#169076,#169077,#169078,#169079,#169080,
#169081,#169082,#169083,#169084,#169085,#169086,#169087,#169088,#169089,
#169090,#169091,#169092,#169093,#169094,#169095,#169096,#169097,#169098,
#169099,#169100,#169101,#169102,#169103,#169104,#169105,#169106,#169107,
#169108,#169109,#169110,#169111,#169112,#169113,#169114,#169115,#169116,
#169117,#169118,#169119,#169120,#169121,#169122,#169123,#169124,#169125,
#169126,#169127,#169128,#169129,#169130,#169131,#169132,#169133,#169134,
#169135,#169136,#169137,#169138,#169139,#169140,#169141,#169142,#169143,
#169144,#169145,#169146,#169147,#169148,#169149,#169150,#169151,#169152,
#169153,#169154,#169155,#169156,#169157,#169158,#169159,#169160,#169161,
#169162,#169163,#169164,#169165,#169166,#169167,#169168,#169169,#169170),
 .UNSPECIFIED.,.F.,.F.,(4,3,3,3,3,3,3,3,3,3,3,3,3,3,3,3,3,3,3,3,3,3,3,3,
3,3,3,3,3,3,3,3,3,3,3,3,3,3,3,3,4),(0.,0.00042823575704742,0.000953028677821348,
0.0296649831518755,0.0591239226216254,0.0715449679712171,0.101238290723875,
0.124999999999999,0.214939059133572,0.246093749999998,0.249999999999998,
0.32793420327691,0.364178809141005,0.374999999999999,0.426885162186684,
0.434050718234393,0.4375,0.46875,0.484375,0.492187500000001,0.496093750000001,
0.498046875000001,0.500000000000001,0.500100116785369,0.582767577315675,
0.625000000000002,0.648830863552705,0.699553986074555,0.716893346557216,
0.738137016722508,0.742187500000003,0.746093750000003,0.750000000000003,
0.785581258945703,0.826685989965252,0.86775510100022,0.908405445427098,
0.930378240366883,0.969699336603254,0.999108385391882,1.),.UNSPECIFIED.);
#24335=B_SPLINE_CURVE_WITH_KNOTS('',3,(#169262,#169263,#169264,#169265),
 .UNSPECIFIED.,.F.,.F.,(4,4),(0.,0.026268696648067),.UNSPECIFIED.);
#24336=B_SPLINE_CURVE_WITH_KNOTS('',3,(#169266,#169267,#169268,#169269),
 .UNSPECIFIED.,.F.,.F.,(4,4),(0.,0.0262686966482326),.UNSPECIFIED.);
#24337=B_SPLINE_CURVE_WITH_KNOTS('',3,(#169493,#169494,#169495,#169496,
#169497,#169498,#169499,#169500,#169501,#169502,#169503,#169504),
 .UNSPECIFIED.,.F.,.F.,(4,2,2,2,2,4),(-0.358600614497163,-0.336590698464702,
-0.314434291168697,-0.269758529940321,-0.179530499588331,0.),
 .UNSPECIFIED.);
#24338=B_SPLINE_CURVE_WITH_KNOTS('',3,(#169506,#169507,#169508,#169509,
#169510,#169511,#169512,#169513,#169514,#169515,#169516,#169517),
 .UNSPECIFIED.,.F.,.F.,(4,2,2,2,2,4),(-0.358600621348355,-0.336590661936306,
-0.314434253593136,-0.269758494188564,-0.179530484335802,0.),
 .UNSPECIFIED.);
#24339=B_SPLINE_CURVE_WITH_KNOTS('',3,(#169518,#169519,#169520,#169521,
#169522,#169523,#169524,#169525,#169526,#169527,#169528,#169529,#169530,
#169531,#169532,#169533,#169534,#169535,#169536,#169537,#169538,#169539,
#169540,#169541,#169542,#169543,#169544,#169545,#169546,#169547,#169548,
#169549,#169550,#169551,#169552,#169553,#169554,#169555,#169556,#169557,
#169558,#169559,#169560,#169561,#169562,#169563,#169564,#169565,#169566,
#169567,#169568,#169569,#169570,#169571,#169572,#169573,#169574,#169575,
#169576,#169577,#169578,#169579,#169580,#169581,#169582,#169583,#169584,
#169585,#169586,#169587,#169588,#169589,#169590,#169591,#169592,#169593,
#169594,#169595,#169596,#169597,#169598,#169599,#169600,#169601,#169602,
#169603,#169604,#169605,#169606,#169607,#169608,#169609,#169610,#169611),
 .UNSPECIFIED.,.F.,.F.,(4,3,3,3,3,3,3,3,3,3,3,3,3,3,3,3,3,3,3,3,3,3,3,3,
3,3,3,3,3,3,3,4),(7.07383405333801E-9,0.000185481200514374,0.00209789788204644,
0.00593407499601808,0.0371456031055623,0.0774279743208184,0.101927509204789,
0.142817818939058,0.168586675415445,0.20952907741012,0.235207511954171,
0.25,0.300771028306561,0.366577698048115,0.438379241599273,0.499951864993755,
0.5,0.578342126744578,0.633450287347176,0.699317094696975,0.75,0.764868961176406,
0.80547318591929,0.831490470403233,0.872074648468611,0.898160396314077,
0.938061990284187,0.962902096319114,0.994062344852343,0.997890509989055,
0.999798786687148,0.999999999553271),.UNSPECIFIED.);
#24340=B_SPLINE_CURVE_WITH_KNOTS('',3,(#169685,#169686,#169687,#169688),
 .UNSPECIFIED.,.F.,.F.,(4,4),(-0.931540742513151,-1.04317168914391E-10),
 .UNSPECIFIED.);
#24341=B_SPLINE_CURVE_WITH_KNOTS('',3,(#169691,#169692,#169693,#169694),
 .UNSPECIFIED.,.F.,.F.,(4,4),(-0.931540739806317,-1.04317110474898E-10),
 .UNSPECIFIED.);
#24342=B_SPLINE_CURVE_WITH_KNOTS('',3,(#169851,#169852,#169853,#169854,
#169855,#169856,#169857,#169858,#169859,#169860),.UNSPECIFIED.,.F.,.F.,
(4,2,2,2,4),(0.,0.133115171967196,0.274762912401081,0.416400475291265,0.54980469291253),
 .UNSPECIFIED.);
#24343=B_SPLINE_CURVE_WITH_KNOTS('',3,(#169861,#169862,#169863,#169864,
#169865,#169866,#169867,#169868,#169869,#169870),.UNSPECIFIED.,.F.,.F.,
(4,2,2,2,4),(0.,0.133115213677724,0.27476292019439,0.416400641733826,0.549804817426638),
 .UNSPECIFIED.);
#24344=B_SPLINE_CURVE_WITH_KNOTS('',3,(#169882,#169883,#169884,#169885),
 .UNSPECIFIED.,.F.,.F.,(4,4),(2.03287907341032E-19,0.0122388605934849),
 .UNSPECIFIED.);
#24345=B_SPLINE_CURVE_WITH_KNOTS('',3,(#169887,#169888,#169889,#169890),
 .UNSPECIFIED.,.F.,.F.,(4,4),(0.,0.0122414931162063),.UNSPECIFIED.);
#24346=B_SPLINE_CURVE_WITH_KNOTS('',3,(#169953,#169954,#169955,#169956,
#169957,#169958,#169959,#169960,#169961,#169962),.UNSPECIFIED.,.F.,.F.,
(4,2,2,2,4),(1.0000000459831E-6,0.156718909328961,0.329756212037607,0.502919854676326,
0.659729926439619),.UNSPECIFIED.);
#26409=LINE('',#168389,#28497);
#26410=LINE('',#168396,#28498);
#26411=LINE('',#168401,#28499);
#26412=LINE('',#168416,#28500);
#26413=LINE('',#168428,#28501);
#26414=LINE('',#168431,#28502);
#26415=LINE('',#168447,#28503);
#26416=LINE('',#168531,#28504);
#26417=LINE('',#168643,#28505);
#26418=LINE('',#168656,#28506);
#26419=LINE('',#168669,#28507);
#26420=LINE('',#168990,#28508);
#26421=LINE('',#168991,#28509);
#26422=LINE('',#169875,#28510);
#26423=LINE('',#169876,#28511);
#26424=LINE('',#169880,#28512);
#26425=LINE('',#169964,#28513);
#28497=VECTOR('',#92241,2.5);
#28498=VECTOR('',#92250,2.50000000008162);
#28499=VECTOR('',#92257,2.5);
#28500=VECTOR('',#92260,1000.);
#28501=VECTOR('',#92261,1000.);
#28502=VECTOR('',#92264,2.50000000013396);
#28503=VECTOR('',#92273,1000.);
#28504=VECTOR('',#92278,1000.);
#28505=VECTOR('',#92279,1000.);
#28506=VECTOR('',#92282,1000.);
#28507=VECTOR('',#92285,1000.);
#28508=VECTOR('',#92286,1000.);
#28509=VECTOR('',#92287,1000.);
#28510=VECTOR('',#92294,1000.);
#28511=VECTOR('',#92295,1000.);
#28512=VECTOR('',#92300,1000.);
#28513=VECTOR('',#92309,1000.);
#33889=VERTEX_POINT('',#168385);
#33890=VERTEX_POINT('',#168386);
#33891=VERTEX_POINT('',#168388);
#33892=VERTEX_POINT('',#168393);
#33893=VERTEX_POINT('',#168395);
#33894=VERTEX_POINT('',#168399);
#33895=VERTEX_POINT('',#168403);
#33896=VERTEX_POINT('',#168404);
#33897=VERTEX_POINT('',#168415);
#33898=VERTEX_POINT('',#168417);
#33899=VERTEX_POINT('',#168430);
#33900=VERTEX_POINT('',#168434);
#33901=VERTEX_POINT('',#168435);
#33902=VERTEX_POINT('',#168437);
#33903=VERTEX_POINT('',#168444);
#33904=VERTEX_POINT('',#168446);
#33905=VERTEX_POINT('',#168448);
#33906=VERTEX_POINT('',#168450);
#33907=VERTEX_POINT('',#168457);
#33908=VERTEX_POINT('',#168519);
#33909=VERTEX_POINT('',#168530);
#33910=VERTEX_POINT('',#168532);
#33911=VERTEX_POINT('',#168642);
#33912=VERTEX_POINT('',#168655);
#33913=VERTEX_POINT('',#168668);
#33914=VERTEX_POINT('',#168830);
#33915=VERTEX_POINT('',#168831);
#33916=VERTEX_POINT('',#168922);
#33917=VERTEX_POINT('',#168923);
#33918=VERTEX_POINT('',#169032);
#33919=VERTEX_POINT('',#169033);
#33920=VERTEX_POINT('',#169038);
#33921=VERTEX_POINT('',#169045);
#33922=VERTEX_POINT('',#169492);
#33923=VERTEX_POINT('',#169505);
#33924=VERTEX_POINT('',#169684);
#33925=VERTEX_POINT('',#169689);
#33926=VERTEX_POINT('',#169872);
#33927=VERTEX_POINT('',#169873);
#33928=VERTEX_POINT('',#169878);
#33929=VERTEX_POINT('',#169951);
#44533=EDGE_CURVE('',#33889,#33890,#21011,.T.);
#44534=EDGE_CURVE('',#33890,#33891,#26409,.T.);
#44535=EDGE_CURVE('',#33891,#33891,#21012,.T.);
#44536=EDGE_CURVE('',#33890,#33889,#21013,.T.);
#44537=EDGE_CURVE('',#33892,#33892,#21014,.T.);
#44538=EDGE_CURVE('',#33892,#33893,#26410,.T.);
#44539=EDGE_CURVE('',#33893,#33893,#21015,.T.);
#44540=EDGE_CURVE('',#33894,#33894,#21016,.T.);
#44541=EDGE_CURVE('',#33894,#33892,#26411,.T.);
#44542=EDGE_CURVE('',#33895,#33896,#24318,.T.);
#44543=EDGE_CURVE('',#33896,#33897,#26412,.T.);
#44544=EDGE_CURVE('',#33898,#33897,#24319,.F.);
#44545=EDGE_CURVE('',#33895,#33898,#26413,.T.);
#44546=EDGE_CURVE('',#33889,#33899,#26414,.T.);
#44547=EDGE_CURVE('',#33899,#33899,#21017,.T.);
#44548=EDGE_CURVE('',#33900,#33901,#21018,.T.);
#44549=EDGE_CURVE('',#33902,#33900,#24320,.F.);
#44550=EDGE_CURVE('',#33903,#33902,#21019,.T.);
#44551=EDGE_CURVE('',#33904,#33903,#26415,.T.);
#44552=EDGE_CURVE('',#33904,#33905,#21020,.T.);
#44553=EDGE_CURVE('',#33906,#33905,#24321,.F.);
#44554=EDGE_CURVE('',#33907,#33906,#21021,.T.);
#44555=EDGE_CURVE('',#33901,#33907,#24322,.T.);
#44556=EDGE_CURVE('',#33897,#33908,#24323,.T.);
#44557=EDGE_CURVE('',#33909,#33908,#26416,.T.);
#44558=EDGE_CURVE('',#33909,#33910,#24324,.T.);
#44559=EDGE_CURVE('',#33911,#33910,#26417,.T.);
#44560=EDGE_CURVE('',#33911,#33898,#24325,.T.);
#44561=EDGE_CURVE('',#33912,#33911,#26418,.T.);
#44562=EDGE_CURVE('',#33912,#33895,#24326,.T.);
#44563=EDGE_CURVE('',#33908,#33913,#26419,.T.);
#44564=EDGE_CURVE('',#33896,#33913,#24327,.T.);
#44565=EDGE_CURVE('',#33914,#33915,#24328,.T.);
#44566=EDGE_CURVE('',#33910,#33914,#24329,.T.);
#44567=EDGE_CURVE('',#33915,#33909,#24330,.T.);
#44568=EDGE_CURVE('',#33916,#33917,#4458,.T.);
#44569=EDGE_CURVE('',#33913,#33916,#26420,.T.);
#44570=EDGE_CURVE('',#33917,#33912,#26421,.T.);
#44571=EDGE_CURVE('',#33918,#33919,#24331,.T.);
#44572=EDGE_CURVE('',#33920,#33919,#24332,.T.);
#44573=EDGE_CURVE('',#33920,#33921,#24333,.T.);
#44574=EDGE_CURVE('',#33921,#33918,#24334,.T.);
#44575=EDGE_CURVE('',#33920,#33915,#24335,.T.);
#44576=EDGE_CURVE('',#33919,#33914,#24336,.T.);
#44577=EDGE_CURVE('',#33916,#33922,#24337,.T.);
#44578=EDGE_CURVE('',#33917,#33923,#24338,.T.);
#44579=EDGE_CURVE('',#33922,#33923,#24339,.T.);
#44580=EDGE_CURVE('',#33923,#33924,#24340,.T.);
#44581=EDGE_CURVE('',#33925,#33924,#21022,.T.);
#44582=EDGE_CURVE('',#33922,#33925,#24341,.T.);
#44583=EDGE_CURVE('',#33907,#33918,#24342,.T.);
#44584=EDGE_CURVE('',#33901,#33921,#24343,.T.);
#44585=EDGE_CURVE('',#33926,#33927,#21023,.T.);
#44586=EDGE_CURVE('',#33926,#33904,#26422,.T.);
#44587=EDGE_CURVE('',#33903,#33927,#26423,.T.);
#44588=EDGE_CURVE('',#33928,#33902,#192,.T.);
#44589=EDGE_CURVE('',#33927,#33928,#26424,.T.);
#44590=EDGE_CURVE('',#33900,#33925,#24344,.T.);
#44591=EDGE_CURVE('',#33924,#33906,#24345,.T.);
#44592=EDGE_CURVE('',#33905,#33929,#193,.T.);
#44593=EDGE_CURVE('',#33928,#33929,#24346,.T.);
#44594=EDGE_CURVE('',#33929,#33926,#26425,.T.);
#65778=ORIENTED_EDGE('',*,*,#44533,.T.);
#65779=ORIENTED_EDGE('',*,*,#44534,.T.);
#65780=ORIENTED_EDGE('',*,*,#44535,.T.);
#65781=ORIENTED_EDGE('',*,*,#44534,.F.);
#65782=ORIENTED_EDGE('',*,*,#44536,.T.);
#65783=ORIENTED_EDGE('',*,*,#44537,.T.);
#65784=ORIENTED_EDGE('',*,*,#44538,.T.);
#65785=ORIENTED_EDGE('',*,*,#44539,.F.);
#65786=ORIENTED_EDGE('',*,*,#44538,.F.);
#65787=ORIENTED_EDGE('',*,*,#44540,.T.);
#65788=ORIENTED_EDGE('',*,*,#44541,.T.);
#65789=ORIENTED_EDGE('',*,*,#44537,.F.);
#65790=ORIENTED_EDGE('',*,*,#44541,.F.);
#65791=ORIENTED_EDGE('',*,*,#44542,.T.);
#65792=ORIENTED_EDGE('',*,*,#44543,.T.);
#65793=ORIENTED_EDGE('',*,*,#44544,.F.);
#65794=ORIENTED_EDGE('',*,*,#44545,.F.);
#65795=ORIENTED_EDGE('',*,*,#44533,.F.);
#65796=ORIENTED_EDGE('',*,*,#44546,.T.);
#65797=ORIENTED_EDGE('',*,*,#44547,.T.);
#65798=ORIENTED_EDGE('',*,*,#44546,.F.);
#65799=ORIENTED_EDGE('',*,*,#44536,.F.);
#65800=ORIENTED_EDGE('',*,*,#44548,.F.);
#65801=ORIENTED_EDGE('',*,*,#44549,.F.);
#65802=ORIENTED_EDGE('',*,*,#44550,.F.);
#65803=ORIENTED_EDGE('',*,*,#44551,.F.);
#65804=ORIENTED_EDGE('',*,*,#44552,.T.);
#65805=ORIENTED_EDGE('',*,*,#44553,.F.);
#65806=ORIENTED_EDGE('',*,*,#44554,.F.);
#65807=ORIENTED_EDGE('',*,*,#44555,.F.);
#65808=ORIENTED_EDGE('',*,*,#44556,.T.);
#65809=ORIENTED_EDGE('',*,*,#44557,.F.);
#65810=ORIENTED_EDGE('',*,*,#44558,.T.);
#65811=ORIENTED_EDGE('',*,*,#44559,.F.);
#65812=ORIENTED_EDGE('',*,*,#44560,.T.);
#65813=ORIENTED_EDGE('',*,*,#44544,.T.);
#65814=ORIENTED_EDGE('',*,*,#44561,.F.);
#65815=ORIENTED_EDGE('',*,*,#44562,.T.);
#65816=ORIENTED_EDGE('',*,*,#44545,.T.);
#65817=ORIENTED_EDGE('',*,*,#44560,.F.);
#65818=ORIENTED_EDGE('',*,*,#44563,.F.);
#65819=ORIENTED_EDGE('',*,*,#44556,.F.);
#65820=ORIENTED_EDGE('',*,*,#44543,.F.);
#65821=ORIENTED_EDGE('',*,*,#44564,.T.);
#65822=ORIENTED_EDGE('',*,*,#44565,.F.);
#65823=ORIENTED_EDGE('',*,*,#44566,.F.);
#65824=ORIENTED_EDGE('',*,*,#44558,.F.);
#65825=ORIENTED_EDGE('',*,*,#44567,.F.);
#65826=ORIENTED_EDGE('',*,*,#44568,.F.);
#65827=ORIENTED_EDGE('',*,*,#44569,.F.);
#65828=ORIENTED_EDGE('',*,*,#44564,.F.);
#65829=ORIENTED_EDGE('',*,*,#44542,.F.);
#65830=ORIENTED_EDGE('',*,*,#44562,.F.);
#65831=ORIENTED_EDGE('',*,*,#44570,.F.);
#65832=ORIENTED_EDGE('',*,*,#44571,.T.);
#65833=ORIENTED_EDGE('',*,*,#44572,.F.);
#65834=ORIENTED_EDGE('',*,*,#44573,.T.);
#65835=ORIENTED_EDGE('',*,*,#44574,.T.);
#65836=ORIENTED_EDGE('',*,*,#44575,.F.);
#65837=ORIENTED_EDGE('',*,*,#44572,.T.);
#65838=ORIENTED_EDGE('',*,*,#44576,.T.);
#65839=ORIENTED_EDGE('',*,*,#44565,.T.);
#65840=ORIENTED_EDGE('',*,*,#44577,.F.);
#65841=ORIENTED_EDGE('',*,*,#44568,.T.);
#65842=ORIENTED_EDGE('',*,*,#44578,.T.);
#65843=ORIENTED_EDGE('',*,*,#44579,.F.);
#65844=ORIENTED_EDGE('',*,*,#44580,.T.);
#65845=ORIENTED_EDGE('',*,*,#44581,.F.);
#65846=ORIENTED_EDGE('',*,*,#44582,.F.);
#65847=ORIENTED_EDGE('',*,*,#44579,.T.);
#65848=ORIENTED_EDGE('',*,*,#44555,.T.);
#65849=ORIENTED_EDGE('',*,*,#44583,.T.);
#65850=ORIENTED_EDGE('',*,*,#44574,.F.);
#65851=ORIENTED_EDGE('',*,*,#44584,.F.);
#65852=ORIENTED_EDGE('',*,*,#44585,.F.);
#65853=ORIENTED_EDGE('',*,*,#44586,.T.);
#65854=ORIENTED_EDGE('',*,*,#44551,.T.);
#65855=ORIENTED_EDGE('',*,*,#44587,.T.);
#65856=ORIENTED_EDGE('',*,*,#44550,.T.);
#65857=ORIENTED_EDGE('',*,*,#44588,.F.);
#65858=ORIENTED_EDGE('',*,*,#44589,.F.);
#65859=ORIENTED_EDGE('',*,*,#44587,.F.);
#65860=ORIENTED_EDGE('',*,*,#44540,.F.);
#65861=ORIENTED_EDGE('',*,*,#44557,.T.);
#65862=ORIENTED_EDGE('',*,*,#44563,.T.);
#65863=ORIENTED_EDGE('',*,*,#44569,.T.);
#65864=ORIENTED_EDGE('',*,*,#44577,.T.);
#65865=ORIENTED_EDGE('',*,*,#44582,.T.);
#65866=ORIENTED_EDGE('',*,*,#44590,.F.);
#65867=ORIENTED_EDGE('',*,*,#44548,.T.);
#65868=ORIENTED_EDGE('',*,*,#44584,.T.);
#65869=ORIENTED_EDGE('',*,*,#44573,.F.);
#65870=ORIENTED_EDGE('',*,*,#44575,.T.);
#65871=ORIENTED_EDGE('',*,*,#44567,.T.);
#65872=ORIENTED_EDGE('',*,*,#44539,.T.);
#65873=ORIENTED_EDGE('',*,*,#44578,.F.);
#65874=ORIENTED_EDGE('',*,*,#44570,.T.);
#65875=ORIENTED_EDGE('',*,*,#44561,.T.);
#65876=ORIENTED_EDGE('',*,*,#44559,.T.);
#65877=ORIENTED_EDGE('',*,*,#44566,.T.);
#65878=ORIENTED_EDGE('',*,*,#44576,.F.);
#65879=ORIENTED_EDGE('',*,*,#44571,.F.);
#65880=ORIENTED_EDGE('',*,*,#44583,.F.);
#65881=ORIENTED_EDGE('',*,*,#44554,.T.);
#65882=ORIENTED_EDGE('',*,*,#44591,.F.);
#65883=ORIENTED_EDGE('',*,*,#44580,.F.);
#65884=ORIENTED_EDGE('',*,*,#44547,.F.);
#65885=ORIENTED_EDGE('',*,*,#44592,.T.);
#65886=ORIENTED_EDGE('',*,*,#44593,.F.);
#65887=ORIENTED_EDGE('',*,*,#44588,.T.);
#65888=ORIENTED_EDGE('',*,*,#44549,.T.);
#65889=ORIENTED_EDGE('',*,*,#44590,.T.);
#65890=ORIENTED_EDGE('',*,*,#44581,.T.);
#65891=ORIENTED_EDGE('',*,*,#44591,.T.);
#65892=ORIENTED_EDGE('',*,*,#44553,.T.);
#65893=ORIENTED_EDGE('',*,*,#44593,.T.);
#65894=ORIENTED_EDGE('',*,*,#44594,.T.);
#65895=ORIENTED_EDGE('',*,*,#44585,.T.);
#65896=ORIENTED_EDGE('',*,*,#44589,.T.);
#65897=ORIENTED_EDGE('',*,*,#44586,.F.);
#65898=ORIENTED_EDGE('',*,*,#44594,.F.);
#65899=ORIENTED_EDGE('',*,*,#44592,.F.);
#65900=ORIENTED_EDGE('',*,*,#44552,.F.);
#65901=ORIENTED_EDGE('',*,*,#44535,.F.);
#66127=CONICAL_SURFACE('',#77686,2.50000000008162,0.78539816269889);
#66128=CONICAL_SURFACE('',#77692,2.50000000013396,0.785398162698949);
#71354=ADVANCED_FACE('',(#10604),#5369,.F.);
#71355=ADVANCED_FACE('',(#10605),#66127,.F.);
#71356=ADVANCED_FACE('',(#10606),#5370,.F.);
#71357=ADVANCED_FACE('',(#10607),#5371,.T.);
#71358=ADVANCED_FACE('',(#10608),#66128,.F.);
#71359=ADVANCED_FACE('',(#10609),#5372,.T.);
#71360=ADVANCED_FACE('',(#10610),#4370,.F.);
#71361=ADVANCED_FACE('',(#10611),#5373,.T.);
#71362=ADVANCED_FACE('',(#10612),#5374,.T.);
#71363=ADVANCED_FACE('',(#10613),#4371,.F.);
#71364=ADVANCED_FACE('',(#10614),#4372,.F.);
#71365=ADVANCED_FACE('',(#10615),#36,.T.);
#71366=ADVANCED_FACE('',(#10616),#37,.T.);
#71367=ADVANCED_FACE('',(#10617),#4373,.T.);
#71368=ADVANCED_FACE('',(#10618),#38,.T.);
#71369=ADVANCED_FACE('',(#10619),#4374,.F.);
#71370=ADVANCED_FACE('',(#10620),#98,.T.);
#71371=ADVANCED_FACE('',(#10621,#76),#99,.F.);
#71372=ADVANCED_FACE('',(#10622,#77),#100,.T.);
#71373=ADVANCED_FACE('',(#10623,#78),#101,.F.);
#71374=ADVANCED_FACE('',(#10624),#39,.T.);
#71375=ADVANCED_FACE('',(#10625),#5375,.F.);
#71376=ADVANCED_FACE('',(#10626,#79),#102,.F.);
#71400=CLOSED_SHELL('',(#71354,#71355,#71356,#71357,#71358,#71359,#71360,
#71361,#71362,#71363,#71364,#71365,#71366,#71367,#71368,#71369,#71370,#71371,
#71372,#71373,#71374,#71375,#71376));
#77681=AXIS2_PLACEMENT_3D('',#168383,#92235,#92236);
#77682=AXIS2_PLACEMENT_3D('',#168384,#92237,#92238);
#77683=AXIS2_PLACEMENT_3D('',#168387,#92239,#92240);
#77684=AXIS2_PLACEMENT_3D('',#168390,#92242,#92243);
#77685=AXIS2_PLACEMENT_3D('',#168391,#92244,#92245);
#77686=AXIS2_PLACEMENT_3D('',#168392,#92246,#92247);
#77687=AXIS2_PLACEMENT_3D('',#168394,#92248,#92249);
#77688=AXIS2_PLACEMENT_3D('',#168397,#92251,#92252);
#77689=AXIS2_PLACEMENT_3D('',#168398,#92253,#92254);
#77690=AXIS2_PLACEMENT_3D('',#168400,#92255,#92256);
#77691=AXIS2_PLACEMENT_3D('',#168402,#92258,#92259);
#77692=AXIS2_PLACEMENT_3D('',#168429,#92262,#92263);
#77693=AXIS2_PLACEMENT_3D('',#168432,#92265,#92266);
#77694=AXIS2_PLACEMENT_3D('',#168433,#92267,#92268);
#77695=AXIS2_PLACEMENT_3D('',#168436,#92269,#92270);
#77696=AXIS2_PLACEMENT_3D('',#168445,#92271,#92272);
#77697=AXIS2_PLACEMENT_3D('',#168449,#92274,#92275);
#77698=AXIS2_PLACEMENT_3D('',#168458,#92276,#92277);
#77699=AXIS2_PLACEMENT_3D('',#168654,#92280,#92281);
#77700=AXIS2_PLACEMENT_3D('',#168667,#92283,#92284);
#77701=AXIS2_PLACEMENT_3D('',#169690,#92288,#92289);
#77702=AXIS2_PLACEMENT_3D('',#169871,#92290,#92291);
#77703=AXIS2_PLACEMENT_3D('',#169874,#92292,#92293);
#77704=AXIS2_PLACEMENT_3D('',#169877,#92296,#92297);
#77705=AXIS2_PLACEMENT_3D('',#169879,#92298,#92299);
#77706=AXIS2_PLACEMENT_3D('',#169881,#92301,#92302);
#77707=AXIS2_PLACEMENT_3D('',#169886,#92303,#92304);
#77708=AXIS2_PLACEMENT_3D('',#169952,#92305,#92306);
#77709=AXIS2_PLACEMENT_3D('',#169963,#92307,#92308);
#77710=AXIS2_PLACEMENT_3D('',#169965,#92310,#92311);
#92235=DIRECTION('axis',(0.,0.,1.));
#92236=DIRECTION('refdir',(1.,0.,0.));
#92237=DIRECTION('center_axis',(0.,6.93889390390723E-16,1.));
#92238=DIRECTION('ref_axis',(0.,-1.,6.93889390390723E-16));
#92239=DIRECTION('center_axis',(0.,0.,-1.));
#92240=DIRECTION('ref_axis',(1.,0.,0.));
#92241=DIRECTION('',(0.,6.93889390390723E-16,1.));
#92242=DIRECTION('center_axis',(0.,6.93889390390723E-16,1.));
#92243=DIRECTION('ref_axis',(0.,-1.,6.93889390390723E-16));
#92244=DIRECTION('center_axis',(0.,0.,-1.));
#92245=DIRECTION('ref_axis',(1.,0.,0.));
#92246=DIRECTION('center_axis',(-3.63153646019851E-17,-6.92938439083296E-16,
1.));
#92247=DIRECTION('ref_axis',(-3.45341426252241E-35,-1.,-6.92938439083296E-16));
#92248=DIRECTION('center_axis',(-1.52446456598325E-14,7.98938021243665E-16,
-1.));
#92249=DIRECTION('ref_axis',(0.998629534767396,-0.0523359559982918,-1.52655665880975E-14));
#92250=DIRECTION('',(-1.12274446152321E-16,0.707106780692592,0.707106781680503));
#92251=DIRECTION('center_axis',(0.,0.,-1.));
#92252=DIRECTION('ref_axis',(1.,0.,0.));
#92253=DIRECTION('center_axis',(0.,-3.46944695195361E-16,1.));
#92254=DIRECTION('ref_axis',(0.,-1.,-3.46944695195361E-16));
#92255=DIRECTION('center_axis',(0.,3.46944695195361E-16,-1.));
#92256=DIRECTION('ref_axis',(0.,-1.,-3.46944695195361E-16));
#92257=DIRECTION('',(0.,-3.46944695195361E-16,1.));
#92258=DIRECTION('center_axis',(-0.743144825477131,-0.669130606359151,0.));
#92259=DIRECTION('ref_axis',(0.669130606359151,-0.743144825477131,0.));
#92260=DIRECTION('',(-0.743144825354978,-0.669130606494815,5.74180650796065E-11));
#92261=DIRECTION('',(-0.743144825338902,-0.669130606512669,-6.51837050591796E-11));
#92262=DIRECTION('center_axis',(1.68138855363801E-15,-1.86737117074379E-15,
-1.));
#92263=DIRECTION('ref_axis',(2.23032315803962E-31,1.,-1.86737117074379E-15));
#92264=DIRECTION('',(1.10232564335427E-15,-0.707106780692635,-0.70710678168046));
#92265=DIRECTION('center_axis',(0.,0.,-1.));
#92266=DIRECTION('ref_axis',(-1.,0.,0.));
#92267=DIRECTION('center_axis',(-3.79384149091044E-17,-3.92183207036316E-16,
-1.));
#92268=DIRECTION('ref_axis',(-0.765634450688746,-0.643275903418232,2.81328964270679E-16));
#92269=DIRECTION('center_axis',(3.79384149091044E-17,3.92183207036316E-16,
1.));
#92270=DIRECTION('ref_axis',(1.57435551588766E-33,1.,-3.92183207036316E-16));
#92271=DIRECTION('center_axis',(-3.79384149091044E-17,-3.92183207036316E-16,
-1.));
#92272=DIRECTION('ref_axis',(-1.16783860824811E-33,1.,-3.92183207036316E-16));
#92273=DIRECTION('',(0.,0.,1.));
#92274=DIRECTION('center_axis',(1.23118896951448E-16,-1.32862593793964E-16,
-1.));
#92275=DIRECTION('ref_axis',(-1.44020741115392E-33,1.,-1.32862593793964E-16));
#92276=DIRECTION('center_axis',(-3.79384149091044E-17,-3.92183207036316E-16,
-1.));
#92277=DIRECTION('ref_axis',(1.57435551588766E-33,1.,-3.92183207036316E-16));
#92278=DIRECTION('',(0.669130606258963,-0.74314482556734,0.));
#92279=DIRECTION('',(-0.669130606258963,0.74314482556734,0.));
#92280=DIRECTION('center_axis',(-0.743144825477572,-0.669130606358661,-5.1412188556418E-14));
#92281=DIRECTION('ref_axis',(0.669130606358661,-0.743144825477572,9.69152791773566E-30));
#92282=DIRECTION('',(-0.743144825477595,-0.669130606358635,0.));
#92283=DIRECTION('center_axis',(-0.743144825477598,-0.669130606358632,9.65978868287187E-15));
#92284=DIRECTION('ref_axis',(0.669130606358632,-0.743144825477598,-7.53421370458092E-30));
#92285=DIRECTION('',(0.743144825477595,0.669130606358636,0.));
#92286=DIRECTION('',(-0.66913060645258,0.743144825393007,0.));
#92287=DIRECTION('',(0.66913060645258,-0.743144825393007,0.));
#92288=DIRECTION('center_axis',(-0.998629535578219,0.0523359405268506,-2.25173431738112E-16));
#92289=DIRECTION('ref_axis',(0.0515611881252755,0.983846374653154,-0.171428571017072));
#92290=DIRECTION('center_axis',(-0.0348994964802897,-0.999390827026856,
0.));
#92291=DIRECTION('ref_axis',(-0.999390827026856,0.0348994964802897,0.));
#92292=DIRECTION('center_axis',(-0.0348994967020073,-0.999390827019113,
-1.98641521842394E-15));
#92293=DIRECTION('ref_axis',(-0.999390827019113,0.0348994967020073,-8.88178419700125E-16));
#92294=DIRECTION('',(0.999390827026856,-0.0348994964802897,0.));
#92295=DIRECTION('',(-0.999390827026856,0.0348994964802897,0.));
#92296=DIRECTION('center_axis',(0.,0.,1.));
#92297=DIRECTION('ref_axis',(1.,0.,0.));
#92298=DIRECTION('center_axis',(4.74434968313444E-6,-6.69147110686511E-5,
0.999999997749956));
#92299=DIRECTION('ref_axis',(0.964891936205745,-0.262647198641797,-2.21527462117478E-5));
#92300=DIRECTION('',(0.034899496686458,0.999390827019656,0.));
#92301=DIRECTION('center_axis',(0.,0.,1.));
#92302=DIRECTION('ref_axis',(1.,0.,0.));
#92303=DIRECTION('center_axis',(0.,0.,1.));
#92304=DIRECTION('ref_axis',(1.,0.,0.));
#92305=DIRECTION('center_axis',(4.74680614066393E-6,-6.69734503770472E-5,
-0.999999997746012));
#92306=DIRECTION('ref_axis',(0.964894998461477,-0.26263594851529,2.21698052188808E-5));
#92307=DIRECTION('center_axis',(0.0348994967020073,0.999390827019113,1.98641521842394E-15));
#92308=DIRECTION('ref_axis',(0.999390827019113,-0.0348994967020073,-6.11038882754296E-11));
#92309=DIRECTION('',(-0.0348994966864581,-0.999390827019656,0.));
#92310=DIRECTION('center_axis',(0.,0.,-1.));
#92311=DIRECTION('ref_axis',(0.,-1.,0.));
#168383=CARTESIAN_POINT('',(0.,0.,0.));
#168384=CARTESIAN_POINT('Origin',(0.0261679780000001,13.199314767,-5.7));
#168385=CARTESIAN_POINT('',(0.0261679780000018,10.699314766933,-5.69999999993301));
#168386=CARTESIAN_POINT('',(0.0261679779999998,15.699314767,-5.7));
#168387=CARTESIAN_POINT('Origin',(0.026167978,13.199314767,-5.7));
#168388=CARTESIAN_POINT('',(0.0261679779999998,15.699314767,-3.));
#168389=CARTESIAN_POINT('',(0.0261679779999998,15.699314767,-5.7));
#168390=CARTESIAN_POINT('Origin',(0.0261679780000001,13.199314767,-3.));
#168391=CARTESIAN_POINT('Origin',(0.026167978,13.199314767,-5.7));
#168392=CARTESIAN_POINT('Origin',(0.0261679780000001,13.199314767,5.7));
#168393=CARTESIAN_POINT('',(0.0261679779999998,15.6993147670816,5.69999999999998));
#168394=CARTESIAN_POINT('Origin',(0.026167978,13.199314767,5.7));
#168395=CARTESIAN_POINT('',(0.0261679779999998,15.9993147666625,6.00000000000001));
#168396=CARTESIAN_POINT('',(0.0261679779999998,15.6993147670816,5.7));
#168397=CARTESIAN_POINT('Origin',(0.026167978,13.199314767,6.));
#168398=CARTESIAN_POINT('Origin',(0.0261679780000001,13.199314767,3.));
#168399=CARTESIAN_POINT('',(0.0261679779999998,15.699314767,3.));
#168400=CARTESIAN_POINT('Origin',(0.0261679780000001,13.199314767,3.));
#168401=CARTESIAN_POINT('',(0.0261679779999998,15.699314767,3.));
#168402=CARTESIAN_POINT('Origin',(35.6555372325844,21.0677405729214,-4.33680868994202E-16));
#168403=CARTESIAN_POINT('',(43.8189844867682,11.730667947175,-3.90000000000325));
#168404=CARTESIAN_POINT('',(43.8189844868826,11.7306679470941,3.89999999937797));
#168405=CARTESIAN_POINT('Ctrl Pts',(43.8189844868367,11.7306679473376,-3.89999999999328));
#168406=CARTESIAN_POINT('Ctrl Pts',(43.9921002135057,11.6184247178878,-3.26642536031861));
#168407=CARTESIAN_POINT('Ctrl Pts',(44.1237435983594,11.5342903200696,-2.6179058686186));
#168408=CARTESIAN_POINT('Ctrl Pts',(44.2980963496193,11.4231842651665,-1.3114086441359));
#168409=CARTESIAN_POINT('Ctrl Pts',(44.3417418637512,11.3956060716702,-0.656384194552197));
#168410=CARTESIAN_POINT('Ctrl Pts',(44.3417382179344,11.3956083818323,0.656451728908009));
#168411=CARTESIAN_POINT('Ctrl Pts',(44.2980910327637,11.4231876412423,1.31146115586157));
#168412=CARTESIAN_POINT('Ctrl Pts',(44.1237385818983,11.5342935290692,2.61793059663588));
#168413=CARTESIAN_POINT('Ctrl Pts',(43.9920969099076,11.6184268598461,3.26643745082936));
#168414=CARTESIAN_POINT('Ctrl Pts',(43.8189844870025,11.7306679472301,3.89999999938663));
#168415=CARTESIAN_POINT('',(41.8585587172852,9.96549265511137,3.89999999906035));
#168416=CARTESIAN_POINT('',(42.899814893435,10.9030439275682,3.89999999977706));
#168417=CARTESIAN_POINT('',(41.8585587171356,9.9654926551616,-3.89999999979706));
#168418=CARTESIAN_POINT('Ctrl Pts',(41.8585587170749,9.96549265526622,3.89999999897544));
#168419=CARTESIAN_POINT('Ctrl Pts',(42.0425841023629,9.84617591879291,3.22649783117755));
#168420=CARTESIAN_POINT('Ctrl Pts',(42.1797151875545,9.75863037516518,2.53619779817488));
#168421=CARTESIAN_POINT('Ctrl Pts',(42.3430786805369,9.65460011496585,1.22769191823626));
#168422=CARTESIAN_POINT('Ctrl Pts',(42.3813156568265,9.63043105679415,0.614404332577125));
#168423=CARTESIAN_POINT('Ctrl Pts',(42.381312885009,9.63043281314897,-0.614474833094867));
#168424=CARTESIAN_POINT('Ctrl Pts',(42.3430726881961,9.65460391064827,-1.22776580224464));
#168425=CARTESIAN_POINT('Ctrl Pts',(42.1797051458808,9.75863679307803,-2.53624838517435));
#168426=CARTESIAN_POINT('Ctrl Pts',(42.0425773519183,9.84618029558489,-3.2265225368096));
#168427=CARTESIAN_POINT('Ctrl Pts',(41.8585587168806,9.96549265539219,-3.89999999968654));
#168428=CARTESIAN_POINT('',(42.7547095826604,10.7723905189662,-3.90000000032325));
#168429=CARTESIAN_POINT('Origin',(0.0261679780000021,13.199314767,-5.7));
#168430=CARTESIAN_POINT('',(0.0261679780000023,10.3993147672851,-5.99999999999998));
#168431=CARTESIAN_POINT('',(0.0261679780000018,10.699314766866,-5.69999999999999));
#168432=CARTESIAN_POINT('Origin',(0.026167978,13.199314767,-6.));
#168433=CARTESIAN_POINT('Origin',(-3.0444397003393E-13,12.7,6.));
#168434=CARTESIAN_POINT('',(0.0871991420266949,18.6993663254969,5.99999999999862));
#168435=CARTESIAN_POINT('',(5.86033332496759,11.41295170178,6.));
#168436=CARTESIAN_POINT('Origin',(-3.0444397003393E-13,12.7,6.));
#168437=CARTESIAN_POINT('',(-0.481485079125861,18.6806498075813,3.0000000012892));
#168438=CARTESIAN_POINT('Ctrl Pts',(0.0871991550143243,18.6993663259332,
5.99999999693977));
#168439=CARTESIAN_POINT('Ctrl Pts',(-0.0465256260974608,18.7013099791932,
5.43225701180379));
#168440=CARTESIAN_POINT('Ctrl Pts',(-0.170111683726753,18.698530803951,
4.85911197841162));
#168441=CARTESIAN_POINT('Ctrl Pts',(-0.354890542940252,18.6900112704791,
3.85702009702669));
#168442=CARTESIAN_POINT('Ctrl Pts',(-0.42398963631069,18.6852786018039,
3.42948219354828));
#168443=CARTESIAN_POINT('Ctrl Pts',(-0.481485043323748,18.6806498107172,
2.99999999710726));
#168444=CARTESIAN_POINT('',(4.74822287554126,9.0319787999811,3.));
#168445=CARTESIAN_POINT('Origin',(-3.04557785278657E-13,12.7,3.));
#168446=CARTESIAN_POINT('',(4.74822287554126,9.0319787999811,-3.));
#168447=CARTESIAN_POINT('',(4.74822287494953,9.03197880000176,3.));
#168448=CARTESIAN_POINT('',(-0.481484270649411,18.6806498727476,-2.99999999903635));
#168449=CARTESIAN_POINT('Origin',(-1.90684057085888E-14,12.7,-3.));
#168450=CARTESIAN_POINT('',(0.087199142033475,18.6993663256232,-6.00000000133027));
#168451=CARTESIAN_POINT('Ctrl Pts',(-0.48148424584236,18.6806498749201,
-2.99999999521028));
#168452=CARTESIAN_POINT('Ctrl Pts',(-0.423989360136962,18.6852786163215,
-3.42948205870502));
#168453=CARTESIAN_POINT('Ctrl Pts',(-0.35489187828681,18.6900111859768,
-3.85701912903971));
#168454=CARTESIAN_POINT('Ctrl Pts',(-0.185541740556634,18.697819402295,
-4.77544283505271));
#168455=CARTESIAN_POINT('Ctrl Pts',(-0.0909082385386381,18.7019550683862,
-5.24382584688238));
#168456=CARTESIAN_POINT('Ctrl Pts',(0.0871991554604803,18.6993663259267,
-5.99999999883431));
#168457=CARTESIAN_POINT('',(5.86033332447927,11.4129517005848,-6.0000000006689));
#168458=CARTESIAN_POINT('Origin',(-3.04899231012839E-13,12.7,-6.));
#168459=CARTESIAN_POINT('Ctrl Pts',(5.86033332441326,11.412951699256,6.));
#168460=CARTESIAN_POINT('Ctrl Pts',(5.86261002860425,11.4233182474286,5.8983154161611));
#168461=CARTESIAN_POINT('Ctrl Pts',(5.86485847361021,11.4336874083783,5.79662961576286));
#168462=CARTESIAN_POINT('Ctrl Pts',(5.868448699,11.450459003,5.632194411));
#168463=CARTESIAN_POINT('Ctrl Pts',(5.869807969,11.456859941,5.569445715));
#168464=CARTESIAN_POINT('Ctrl Pts',(5.871830748,11.466462662,5.475322));
#168465=CARTESIAN_POINT('Ctrl Pts',(5.87250232,11.469663788,5.443947316));
#168466=CARTESIAN_POINT('Ctrl Pts',(5.873505647,11.474465796,5.39688512));
#168467=CARTESIAN_POINT('Ctrl Pts',(5.873839418,11.476066519,5.381197693));
#168468=CARTESIAN_POINT('Ctrl Pts',(5.874339066,11.478467682,5.357666509));
#168469=CARTESIAN_POINT('Ctrl Pts',(5.874505448,11.479268083,5.349822774));
#168470=CARTESIAN_POINT('Ctrl Pts',(5.874754768,11.480468704,5.338057161));
#168471=CARTESIAN_POINT('Ctrl Pts',(5.874837833,11.480868914,5.334135288));
#168472=CARTESIAN_POINT('Ctrl Pts',(5.874962367,11.481469234,5.328252476));
#168473=CARTESIAN_POINT('Ctrl Pts',(5.87500386,11.481669303,5.326291527));
#168474=CARTESIAN_POINT('Ctrl Pts',(5.875086766,11.482069161,5.322369546));
#168475=CARTESIAN_POINT('Ctrl Pts',(5.875128186,11.482268981,5.320408522));
#168476=CARTESIAN_POINT('Ctrl Pts',(5.880467048,11.508031537,5.067432231));
#168477=CARTESIAN_POINT('Ctrl Pts',(5.885220146,11.531803076,4.815812574));
#168478=CARTESIAN_POINT('Ctrl Pts',(5.898038406,11.597664362,4.059816839));
#168479=CARTESIAN_POINT('Ctrl Pts',(5.904669074,11.634275422,3.5546825));
#168480=CARTESIAN_POINT('Ctrl Pts',(5.914950781,11.692903678,2.542161979));
#168481=CARTESIAN_POINT('Ctrl Pts',(5.918600378,11.714915645,2.03477498));
#168482=CARTESIAN_POINT('Ctrl Pts',(5.922211942,11.736952169,1.272010148));
#168483=CARTESIAN_POINT('Ctrl Pts',(5.923102816,11.742468341,1.017360989));
#168484=CARTESIAN_POINT('Ctrl Pts',(5.924286082,11.749816719,0.508071237));
#168485=CARTESIAN_POINT('Ctrl Pts',(5.924578584,11.751649539,0.253521895));
#168486=CARTESIAN_POINT('Ctrl Pts',(5.924576429,11.751636075,-0.509840295));
#168487=CARTESIAN_POINT('Ctrl Pts',(5.923413308,11.744282385,-1.01836763));
#168488=CARTESIAN_POINT('Ctrl Pts',(5.919803707,11.722258,-1.780587582));
#168489=CARTESIAN_POINT('Ctrl Pts',(5.918286894,11.713083094,-2.034565643));
#168490=CARTESIAN_POINT('Ctrl Pts',(5.91457177,11.691057231,-2.542330331));
#168491=CARTESIAN_POINT('Ctrl Pts',(5.912372151,11.678198728,-2.796229212));
#168492=CARTESIAN_POINT('Ctrl Pts',(5.904645385,11.634142573,-3.556755763));
#168493=CARTESIAN_POINT('Ctrl Pts',(5.898005992,11.597492508,-4.061961581));
#168494=CARTESIAN_POINT('Ctrl Pts',(5.885197279,11.531688249,-4.817044188));
#168495=CARTESIAN_POINT('Ctrl Pts',(5.880449993,11.50794786,-5.068283718));
#168496=CARTESIAN_POINT('Ctrl Pts',(5.875073803,11.48200658,-5.322984668));
#168497=CARTESIAN_POINT('Ctrl Pts',(5.874990938,11.481606943,-5.326903007));
#168498=CARTESIAN_POINT('Ctrl Pts',(5.874825036,11.480807249,-5.334739577));
#168499=CARTESIAN_POINT('Ctrl Pts',(5.874742043,11.480407405,-5.338657861));
#168500=CARTESIAN_POINT('Ctrl Pts',(5.874492938,11.479207884,-5.35041271));
#168501=CARTESIAN_POINT('Ctrl Pts',(5.8743267,11.478408216,-5.35824927));
#168502=CARTESIAN_POINT('Ctrl Pts',(5.873827484,11.47600925,-5.381758936));
#168503=CARTESIAN_POINT('Ctrl Pts',(5.873494003,11.474409991,-5.397432027));
#168504=CARTESIAN_POINT('Ctrl Pts',(5.872491546,11.469612372,-5.44445124));
#168505=CARTESIAN_POINT('Ctrl Pts',(5.871820559,11.466414169,-5.475797302));
#168506=CARTESIAN_POINT('Ctrl Pts',(5.869799547,11.456820204,-5.569835256));
#168507=CARTESIAN_POINT('Ctrl Pts',(5.868441471,11.450425087,-5.632526913));
#168508=CARTESIAN_POINT('Ctrl Pts',(5.86485441801766,11.4336687031271,-5.79681304737971));
#168509=CARTESIAN_POINT('Ctrl Pts',(5.86260797772381,11.4233089067647,-5.8984070333042));
#168510=CARTESIAN_POINT('Ctrl Pts',(5.86033332291787,11.4129516980425,-6.00000000037477));
#168511=CARTESIAN_POINT('Ctrl Pts',(42.0911037142801,9.36912484717797,6.00000101283007));
#168512=CARTESIAN_POINT('Ctrl Pts',(39.3678508886227,12.3936035172147,6.00000101283007));
#168513=CARTESIAN_POINT('Ctrl Pts',(42.4790155504863,9.71840223321708,2.01993501455923));
#168514=CARTESIAN_POINT('Ctrl Pts',(39.7557627238316,12.7428809032538,2.01993501455923));
#168515=CARTESIAN_POINT('Ctrl Pts',(42.479015550558,9.71840223328166,-2.01993501234435));
#168516=CARTESIAN_POINT('Ctrl Pts',(39.7557627239033,12.7428809033184,-2.01993501234435));
#168517=CARTESIAN_POINT('Ctrl Pts',(42.091103714491,9.36912484736789,-6.00000101066592));
#168518=CARTESIAN_POINT('Ctrl Pts',(39.3678508888336,12.3936035174046,-6.00000101066592));
#168519=CARTESIAN_POINT('',(39.775504930057,11.9408580355491,5.99999999959819));
#168520=CARTESIAN_POINT('Ctrl Pts',(41.8585587171188,9.96549265521474,3.89999999899657));
#168521=CARTESIAN_POINT('Ctrl Pts',(41.7915034664367,10.0089693400172,4.14541101470715));
#168522=CARTESIAN_POINT('Ctrl Pts',(41.7027507173744,10.0749332406404,4.37982730885032));
#168523=CARTESIAN_POINT('Ctrl Pts',(41.437560283558,10.2895240148895,4.91537047100115));
#168524=CARTESIAN_POINT('Ctrl Pts',(41.2418079413878,10.460439951812,5.19304888977805));
#168525=CARTESIAN_POINT('Ctrl Pts',(40.8236778904308,10.850802708163,5.61258586872592));
#168526=CARTESIAN_POINT('Ctrl Pts',(40.610008609833,11.0595809772413,5.76374643619597));
#168527=CARTESIAN_POINT('Ctrl Pts',(40.1857028808254,11.4944486152704,5.95378049605652));
#168528=CARTESIAN_POINT('Ctrl Pts',(39.9789697604729,11.7148874485651,5.99999999926869));
#168529=CARTESIAN_POINT('Ctrl Pts',(39.7755049300962,11.9408580355844,5.99999999919638));
#168530=CARTESIAN_POINT('',(39.5935147935475,12.1429785621987,5.99999995227989));
#168531=CARTESIAN_POINT('',(39.5935147984967,12.1429785532113,6.));
#168532=CARTESIAN_POINT('',(39.5935148013839,12.1429785439757,-6.00000000014651));
#168533=CARTESIAN_POINT('Ctrl Pts',(39.5935148013912,12.1429785692612,5.99999985683968));
#168534=CARTESIAN_POINT('Ctrl Pts',(39.593592075,12.1435858512692,5.99646324807023));
#168535=CARTESIAN_POINT('Ctrl Pts',(39.5936896902506,12.1442118064789,5.99271350326619));
#168536=CARTESIAN_POINT('Ctrl Pts',(39.5937765000117,12.144828628235,5.98906773188485));
#168537=CARTESIAN_POINT('Ctrl Pts',(39.5938699396201,12.1454925579887,5.98514352514079));
#168538=CARTESIAN_POINT('Ctrl Pts',(39.5939626032986,12.1461563824849,5.98122029151821));
#168539=CARTESIAN_POINT('Ctrl Pts',(39.5940544909761,12.146820102571,5.97729802528116));
#168540=CARTESIAN_POINT('Ctrl Pts',(39.5944224915473,12.1494782323389,5.96158975780617));
#168541=CARTESIAN_POINT('Ctrl Pts',(39.5947780568862,12.1521346914483,5.94589701242429));
#168542=CARTESIAN_POINT('Ctrl Pts',(39.5951212720585,12.1547895263954,5.93021947088647));
#168543=CARTESIAN_POINT('Ctrl Pts',(39.5952931292047,12.156118874263,5.92236930060117));
#168544=CARTESIAN_POINT('Ctrl Pts',(39.5954610237497,12.1574487481375,5.91452309125952));
#168545=CARTESIAN_POINT('Ctrl Pts',(39.5956281799399,12.1587756919312,5.90668024908748));
#168546=CARTESIAN_POINT('Ctrl Pts',(39.5957954963177,12.1601039073498,5.89882989103356));
#168547=CARTESIAN_POINT('Ctrl Pts',(39.5959623996781,12.1614288363532,5.89098285012388));
#168548=CARTESIAN_POINT('Ctrl Pts',(39.5961288904336,12.1627504920826,5.88313908742715));
#168549=CARTESIAN_POINT('Ctrl Pts',(39.5974664033537,12.1733680882849,5.82012577528396));
#168550=CARTESIAN_POINT('Ctrl Pts',(39.5987773377349,12.1837745082137,5.75732404899093));
#168551=CARTESIAN_POINT('Ctrl Pts',(39.6000625634968,12.1939769494452,5.69471380270722));
#168552=CARTESIAN_POINT('Ctrl Pts',(39.6026595696063,12.2145926288025,5.56819969372396));
#168553=CARTESIAN_POINT('Ctrl Pts',(39.6051517709515,12.2343767961233,5.44246194528457));
#168554=CARTESIAN_POINT('Ctrl Pts',(39.6075453455177,12.2533801427068,5.31735075584711));
#168555=CARTESIAN_POINT('Ctrl Pts',(39.6114116087659,12.2840756311731,5.11526271543155));
#168556=CARTESIAN_POINT('Ctrl Pts',(39.6150182208478,12.3127158898712,4.91494819176507));
#168557=CARTESIAN_POINT('Ctrl Pts',(39.6183889244826,12.3394911559076,4.71569049103997));
#168558=CARTESIAN_POINT('Ctrl Pts',(39.6192601312818,12.3464116082377,4.66418947449));
#168559=CARTESIAN_POINT('Ctrl Pts',(39.6201155446289,12.3532072031859,4.61275903935556));
#168560=CARTESIAN_POINT('Ctrl Pts',(39.620955504257,12.3598806685914,4.5613867724762));
#168561=CARTESIAN_POINT('Ctrl Pts',(39.6242419008288,12.3859910352066,4.36038944341434));
#168562=CARTESIAN_POINT('Ctrl Pts',(39.6272921168251,12.4102367492395,4.16028291618282));
#168563=CARTESIAN_POINT('Ctrl Pts',(39.6301229565858,12.4327441129628,3.96032108945468));
#168564=CARTESIAN_POINT('Ctrl Pts',(39.6329590026703,12.4552928709844,3.75999150399772));
#168565=CARTESIAN_POINT('Ctrl Pts',(39.6355748578746,12.476096858426,3.55980715906955));
#168566=CARTESIAN_POINT('Ctrl Pts',(39.6379808835292,12.4952314004158,3.35901407164543));
#168567=CARTESIAN_POINT('Ctrl Pts',(39.6392292102487,12.5051590418709,3.25483589065287));
#168568=CARTESIAN_POINT('Ctrl Pts',(39.6404209470369,12.51463644471,3.15049378121363));
#168569=CARTESIAN_POINT('Ctrl Pts',(39.6415568549947,12.5236686576725,3.0458820293338));
#168570=CARTESIAN_POINT('Ctrl Pts',(39.6417868028536,12.5254970963389,3.02470491881986));
#168571=CARTESIAN_POINT('Ctrl Pts',(39.6420144594068,12.5273073143591,3.00351675988397));
#168572=CARTESIAN_POINT('Ctrl Pts',(39.6422398267747,12.5290993285967,2.98231667365158));
#168573=CARTESIAN_POINT('Ctrl Pts',(39.6465168551583,12.5631082262811,2.5799808280661));
#168574=CARTESIAN_POINT('Ctrl Pts',(39.6499129052792,12.5901115475324,2.17860979623499));
#168575=CARTESIAN_POINT('Ctrl Pts',(39.6524433523305,12.610231922441,1.77858172671342));
#168576=CARTESIAN_POINT('Ctrl Pts',(39.6549216196748,12.6299374002015,1.3868025345575));
#168577=CARTESIAN_POINT('Ctrl Pts',(39.6565696544995,12.6430411851066,0.996314889485204));
#168578=CARTESIAN_POINT('Ctrl Pts',(39.6574078822912,12.6497060239315,0.607453803531702));
#168579=CARTESIAN_POINT('Ctrl Pts',(39.6577121126954,12.6521249924141,0.466318700987944));
#168580=CARTESIAN_POINT('Ctrl Pts',(39.6579097212539,12.6536961879894,0.32539765540149));
#168581=CARTESIAN_POINT('Ctrl Pts',(39.6580018598091,12.6544287847528,0.184705849465022));
#168582=CARTESIAN_POINT('Ctrl Pts',(39.6580386759582,12.6547215111974,0.128489095319149));
#168583=CARTESIAN_POINT('Ctrl Pts',(39.6580585448889,12.6548794892148,0.0732962827061743));
#168584=CARTESIAN_POINT('Ctrl Pts',(39.6580618011315,12.6549058756015,0.0164255705731008));
#168585=CARTESIAN_POINT('Ctrl Pts',(39.6580621134569,12.6549084064748,0.0109707664936554));
#168586=CARTESIAN_POINT('Ctrl Pts',(39.6580622680239,12.6549096875733,0.00550052285318253));
#168587=CARTESIAN_POINT('Ctrl Pts',(39.6580622619614,12.654909696507,1.24535000317211E-5));
#168588=CARTESIAN_POINT('Ctrl Pts',(39.6580622573028,12.6549097033719,-0.00420478650620587));
#168589=CARTESIAN_POINT('Ctrl Pts',(39.6580621581765,12.6549089583405,-0.00842206125982745));
#168590=CARTESIAN_POINT('Ctrl Pts',(39.6580619645721,12.654907461339,-0.0126393699191901));
#168591=CARTESIAN_POINT('Ctrl Pts',(39.6580434310409,12.6547641550369,-0.416357675171431));
#168592=CARTESIAN_POINT('Ctrl Pts',(39.6571585579766,12.6477254839266,-0.82038760970862));
#168593=CARTESIAN_POINT('Ctrl Pts',(39.6554014196392,12.6337528094906,-1.22436402282335));
#168594=CARTESIAN_POINT('Ctrl Pts',(39.6549935243686,12.6305092471041,-1.3181415386889));
#168595=CARTESIAN_POINT('Ctrl Pts',(39.6545386527295,12.6268922498283,-1.41191618938065));
#168596=CARTESIAN_POINT('Ctrl Pts',(39.6540367805458,12.6229017314022,-1.50568344113572));
#168597=CARTESIAN_POINT('Ctrl Pts',(39.6518789316225,12.6057441040828,-1.90884498271349));
#168598=CARTESIAN_POINT('Ctrl Pts',(39.6488521168538,12.5816768701136,-2.3118683700991));
#168599=CARTESIAN_POINT('Ctrl Pts',(39.6449594170072,12.550724154806,-2.71439124863566));
#168600=CARTESIAN_POINT('Ctrl Pts',(39.64415731637,12.5443462696235,-2.79733210461966));
#168601=CARTESIAN_POINT('Ctrl Pts',(39.6433184742028,12.537676217345,-2.88025173026906));
#168602=CARTESIAN_POINT('Ctrl Pts',(39.6424429513847,12.5307144788084,-2.96314699548041));
#168603=CARTESIAN_POINT('Ctrl Pts',(39.642277643315,12.5294000281332,-2.97879850792345));
#168604=CARTESIAN_POINT('Ctrl Pts',(39.6420987002013,12.5279771573245,-2.99559802050964));
#168605=CARTESIAN_POINT('Ctrl Pts',(39.641943068,12.5267399763259,-3.01009890988096));
#168606=CARTESIAN_POINT('Ctrl Pts',(39.6418152351274,12.5257237830207,-3.02200962198725));
#168607=CARTESIAN_POINT('Ctrl Pts',(39.6416865140263,12.5247005122664,-3.03393218069561));
#168608=CARTESIAN_POINT('Ctrl Pts',(39.6415569002152,12.5236701289684,-3.04586656515235));
#168609=CARTESIAN_POINT('Ctrl Pts',(39.6366369001502,12.484557893538,-3.49888288974479));
#168610=CARTESIAN_POINT('Ctrl Pts',(39.6304319642937,12.4351816259025,-3.96893688438699));
#168611=CARTESIAN_POINT('Ctrl Pts',(39.6226760900002,12.3735511564761,-4.45488827013432));
#168612=CARTESIAN_POINT('Ctrl Pts',(39.6221096259592,12.3690498657854,-4.49038059185758));
#168613=CARTESIAN_POINT('Ctrl Pts',(39.6215362581397,12.3644940511062,-4.52587230177962));
#168614=CARTESIAN_POINT('Ctrl Pts',(39.6209556744651,12.3598812745533,-4.56138140435976));
#168615=CARTESIAN_POINT('Ctrl Pts',(39.6187047513006,12.3419975378079,-4.69905021084013));
#168616=CARTESIAN_POINT('Ctrl Pts',(39.6163459195903,12.3232611011816,-4.83698069681983));
#168617=CARTESIAN_POINT('Ctrl Pts',(39.6138572018242,12.3034969681751,-4.97621973194427));
#168618=CARTESIAN_POINT('Ctrl Pts',(39.6118433777902,12.287504200091,-5.08888936416476));
#168619=CARTESIAN_POINT('Ctrl Pts',(39.609744395501,12.2708376377433,-5.20241573595815));
#168620=CARTESIAN_POINT('Ctrl Pts',(39.6075454849006,12.2533798111742,-5.31735177347078));
#168621=CARTESIAN_POINT('Ctrl Pts',(39.6051735931911,12.2345486344544,-5.44132945335634));
#168622=CARTESIAN_POINT('Ctrl Pts',(39.6026865372115,12.2148054121144,-5.56689293064617));
#168623=CARTESIAN_POINT('Ctrl Pts',(39.6000626637871,12.1939767452097,-5.69471430525968));
#168624=CARTESIAN_POINT('Ctrl Pts',(39.5987849050625,12.1838337213083,-5.75696001996335));
#168625=CARTESIAN_POINT('Ctrl Pts',(39.5974746226702,12.1734326499498,-5.81974212209882));
#168626=CARTESIAN_POINT('Ctrl Pts',(39.5961289372154,12.1627504039713,-5.88313927508247));
#168627=CARTESIAN_POINT('Ctrl Pts',(39.5959625743245,12.1614297912558,-5.89097686715119));
#168628=CARTESIAN_POINT('Ctrl Pts',(39.5957956701409,12.1601048790975,-5.89882385904714));
#168629=CARTESIAN_POINT('Ctrl Pts',(39.5956282185228,12.1587756206009,-5.90668039857604));
#168630=CARTESIAN_POINT('Ctrl Pts',(39.5954611918017,12.1574497350065,-5.91451700267563));
#168631=CARTESIAN_POINT('Ctrl Pts',(39.5952932983793,12.1561198748105,-5.92236316287808));
#168632=CARTESIAN_POINT('Ctrl Pts',(39.59512130112,12.154789472191,-5.93021958221744));
#168633=CARTESIAN_POINT('Ctrl Pts',(39.5947786320197,12.1521389190903,-5.94587187899884));
#168634=CARTESIAN_POINT('Ctrl Pts',(39.5944231052091,12.1494825187348,-5.96156430842148));
#168635=CARTESIAN_POINT('Ctrl Pts',(39.5940545004811,12.1468200840298,-5.97729806109937));
#168636=CARTESIAN_POINT('Ctrl Pts',(39.5939626487262,12.1461566381176,-5.98121871833759));
#168637=CARTESIAN_POINT('Ctrl Pts',(39.5938699849262,12.145492817321,-5.98514194177266));
#168638=CARTESIAN_POINT('Ctrl Pts',(39.5937765051849,12.1448286191576,-5.98906774952607));
#168639=CARTESIAN_POINT('Ctrl Pts',(39.5936897256473,12.1442120277047,-5.99271217319373));
#168640=CARTESIAN_POINT('Ctrl Pts',(39.5935921036083,12.1435860636139,-5.99646200266368));
#168641=CARTESIAN_POINT('Ctrl Pts',(39.5935147981916,12.1429785445163,-6.0000000001696));
#168642=CARTESIAN_POINT('',(39.7755049294992,11.9408580361687,-5.99999999959826));
#168643=CARTESIAN_POINT('',(39.775504929821,11.9408580357326,-6.));
#168644=CARTESIAN_POINT('Ctrl Pts',(39.7755049295383,11.9408580362039,-5.99999999919652));
#168645=CARTESIAN_POINT('Ctrl Pts',(39.9785184064207,11.7153887280077,-5.999999999353));
#168646=CARTESIAN_POINT('Ctrl Pts',(40.1847882503583,11.4954233907689,-5.95398529746107));
#168647=CARTESIAN_POINT('Ctrl Pts',(40.6081030675166,11.0614933541335,-5.76482235717356));
#168648=CARTESIAN_POINT('Ctrl Pts',(40.821279662875,10.8531281619462,-5.61439945620298));
#168649=CARTESIAN_POINT('Ctrl Pts',(41.2398722620509,10.4621498268799,-5.19565760275282));
#168650=CARTESIAN_POINT('Ctrl Pts',(41.4363530791327,10.2905364126708,-4.91747536111852));
#168651=CARTESIAN_POINT('Ctrl Pts',(41.702384420184,10.0752054541128,-4.38079376061105));
#168652=CARTESIAN_POINT('Ctrl Pts',(41.7913649514247,10.0090591491603,-4.14591795633693));
#168653=CARTESIAN_POINT('Ctrl Pts',(41.8585587169246,9.96549265534065,-3.89999999970769));
#168654=CARTESIAN_POINT('Origin',(41.9168260374617,13.8689122198355,-3.00000000000006));
#168655=CARTESIAN_POINT('',(41.7359306988266,13.7060333280929,-5.99999999959819));
#168656=CARTESIAN_POINT('',(41.7359306985475,13.7060333266355,-6.));
#168657=CARTESIAN_POINT('Ctrl Pts',(41.7359306988658,13.7060333281281,-5.99999999919639));
#168658=CARTESIAN_POINT('Ctrl Pts',(41.9400453487107,13.479341043567,-5.99999999940487));
#168659=CARTESIAN_POINT('Ctrl Pts',(42.1474454711246,13.2582206593349,-5.95348484309781));
#168660=CARTESIAN_POINT('Ctrl Pts',(42.5706384879709,12.8246056488402,-5.76333393612528));
#168661=CARTESIAN_POINT('Ctrl Pts',(42.7826771038137,12.6173958832382,-5.61342743869922));
#168662=CARTESIAN_POINT('Ctrl Pts',(43.1952883029083,12.2320043595518,-5.20066911826413));
#168663=CARTESIAN_POINT('Ctrl Pts',(43.3879766152324,12.0634062250566,-4.92990914760786));
#168664=CARTESIAN_POINT('Ctrl Pts',(43.6569747522941,11.8447245299816,-4.39611142481161));
#168665=CARTESIAN_POINT('Ctrl Pts',(43.7495964127534,11.7756569415571,-4.15395117442176));
#168666=CARTESIAN_POINT('Ctrl Pts',(43.8189870849516,11.7306662627757,-3.89999049146802));
#168667=CARTESIAN_POINT('Origin',(41.9168260374619,13.8689122198355,3.00000000000002));
#168668=CARTESIAN_POINT('',(41.7359306996812,13.7060333271437,5.99999999959818));
#168669=CARTESIAN_POINT('',(39.7755049300089,11.9408580353737,6.));
#168670=CARTESIAN_POINT('Ctrl Pts',(43.8189844870475,11.7306679471774,3.89999999940828));
#168671=CARTESIAN_POINT('Ctrl Pts',(43.7497368818761,11.7755660912359,4.1534346662405));
#168672=CARTESIAN_POINT('Ctrl Pts',(43.6573576179347,11.8444391213823,4.39511093543262));
#168673=CARTESIAN_POINT('Ctrl Pts',(43.3892130900103,12.0623655059657,4.92778647249781));
#168674=CARTESIAN_POINT('Ctrl Pts',(43.1972403553305,12.2302769996148,5.19805904759368));
#168675=CARTESIAN_POINT('Ctrl Pts',(42.7850817396402,12.6150648732738,5.61160449838341));
#168676=CARTESIAN_POINT('Ctrl Pts',(42.572559062314,12.822679247634,5.76224353382663));
#168677=CARTESIAN_POINT('Ctrl Pts',(42.1483768580881,13.2572282605142,5.95327516155663));
#168678=CARTESIAN_POINT('Ctrl Pts',(41.9405049600971,13.4788305934348,5.99999999927515));
#168679=CARTESIAN_POINT('Ctrl Pts',(41.7359306997204,13.706033327179,5.99999999919635));
#168680=CARTESIAN_POINT('Ctrl Pts',(39.592093664,12.131166347,6.068318707));
#168681=CARTESIAN_POINT('Ctrl Pts',(39.076055002,12.687534913,6.153779637));
#168682=CARTESIAN_POINT('Ctrl Pts',(38.316324576,12.76466494,6.151311746));
#168683=CARTESIAN_POINT('Ctrl Pts',(39.59240577,12.133760521,6.053314685));
#168684=CARTESIAN_POINT('Ctrl Pts',(39.076369283,12.690126742,6.138775261));
#168685=CARTESIAN_POINT('Ctrl Pts',(38.31664227,12.767258547,6.136307738));
#168686=CARTESIAN_POINT('Ctrl Pts',(39.592717877,12.136354695,6.038310664));
#168687=CARTESIAN_POINT('Ctrl Pts',(39.076683564,12.692718572,6.123770877));
#168688=CARTESIAN_POINT('Ctrl Pts',(38.316959963,12.769852155,6.121303731));
#168689=CARTESIAN_POINT('Ctrl Pts',(39.593186037,12.140245955,6.015804631));
#168690=CARTESIAN_POINT('Ctrl Pts',(39.077154985,12.696606319,6.101264295));
#168691=CARTESIAN_POINT('Ctrl Pts',(38.317436504,12.773742566,6.09879772));
#168692=CARTESIAN_POINT('Ctrl Pts',(39.593338947,12.141540209,6.008334889));
#168693=CARTESIAN_POINT('Ctrl Pts',(39.077309654,12.697899291,6.093780344));
#168694=CARTESIAN_POINT('Ctrl Pts',(38.317595353,12.775039369,6.091295716));
#168695=CARTESIAN_POINT('Ctrl Pts',(39.593577743,12.143490089,5.99703347));
#168696=CARTESIAN_POINT('Ctrl Pts',(39.077549071,12.699847579,6.08249969100001));
#168697=CARTESIAN_POINT('Ctrl Pts',(38.317833619,12.776984575,6.08004271));
#168698=CARTESIAN_POINT('Ctrl Pts',(39.593683639,12.144164263,5.99299088));
#168699=CARTESIAN_POINT('Ctrl Pts',(39.07764945,12.700522186,6.078583732));
#168700=CARTESIAN_POINT('Ctrl Pts',(38.317912503,12.777633031,6.076291707));
#168701=CARTESIAN_POINT('Ctrl Pts',(39.593870468,12.1454918,5.9851444));
#168702=CARTESIAN_POINT('Ctrl Pts',(39.077830235,12.701849801,6.07088678500001));
#168703=CARTESIAN_POINT('Ctrl Pts',(38.318068603,12.778930113,6.068789696));
#168704=CARTESIAN_POINT('Ctrl Pts',(39.59396313,12.146155627,5.981221165));
#168705=CARTESIAN_POINT('Ctrl Pts',(39.077919885,12.702513685,6.067038314));
#168706=CARTESIAN_POINT('Ctrl Pts',(38.318145913,12.779578729,6.065038689));
#168707=CARTESIAN_POINT('Ctrl Pts',(39.594422671,12.149475055,5.961605011));
#168708=CARTESIAN_POINT('Ctrl Pts',(39.078364424,12.7058335,6.047795871));
#168709=CARTESIAN_POINT('Ctrl Pts',(38.318528768,12.782822185,6.046283644));
#168710=CARTESIAN_POINT('Ctrl Pts',(39.594778254,12.152131539,5.945912161));
#168711=CARTESIAN_POINT('Ctrl Pts',(39.078708173,12.708490553,6.03240203800001));
#168712=CARTESIAN_POINT('Ctrl Pts',(38.318823224,12.785418148,6.031279577));
#168713=CARTESIAN_POINT('Ctrl Pts',(39.595293565,12.156117675,5.922372994));
#168714=CARTESIAN_POINT('Ctrl Pts',(39.079205987,12.71247794,6.009311436));
#168715=CARTESIAN_POINT('Ctrl Pts',(38.319247178,12.789313893,6.008773432));
#168716=CARTESIAN_POINT('Ctrl Pts',(39.595461458,12.157447556,5.914526772));
#168717=CARTESIAN_POINT('Ctrl Pts',(39.079367313,12.713800705,6.001658908));
#168718=CARTESIAN_POINT('Ctrl Pts',(38.3193833,12.790600397,6.001348676));
#168719=CARTESIAN_POINT('Ctrl Pts',(39.595795923,12.160102727,5.898833554));
#168720=CARTESIAN_POINT('Ctrl Pts',(39.079699563,12.716547187,5.985742981));
#168721=CARTESIAN_POINT('Ctrl Pts',(38.319673324,12.793353081,5.985433552));
#168722=CARTESIAN_POINT('Ctrl Pts',(39.595962823,12.161427665,5.890986501));
#168723=CARTESIAN_POINT('Ctrl Pts',(39.079865358,12.71791769,5.97778454500001));
#168724=CARTESIAN_POINT('Ctrl Pts',(38.319818049,12.794726679,5.977475519));
#168725=CARTESIAN_POINT('Ctrl Pts',(39.597461918,12.173328269,5.820359025));
#168726=CARTESIAN_POINT('Ctrl Pts',(39.081354587,12.730227887,5.906152583));
#168727=CARTESIAN_POINT('Ctrl Pts',(38.321117997,12.807064359,5.905848986));
#168728=CARTESIAN_POINT('Ctrl Pts',(39.598773123,12.183737104,5.757550619));
#168729=CARTESIAN_POINT('Ctrl Pts',(39.082657224,12.740994793,5.842451083));
#168730=CARTESIAN_POINT('Ctrl Pts',(38.322255163,12.817855555,5.842150827));
#168731=CARTESIAN_POINT('Ctrl Pts',(39.602642674,12.214455312,5.56903997));
#168732=CARTESIAN_POINT('Ctrl Pts',(39.086501869,12.77277097,5.651250253));
#168733=CARTESIAN_POINT('Ctrl Pts',(38.325611506,12.849702405,5.650965805));
#168734=CARTESIAN_POINT('Ctrl Pts',(39.605137062,12.234257258,5.443246713));
#168735=CARTESIAN_POINT('Ctrl Pts',(39.088980476,12.793254628,5.52366008399999));
#168736=CARTESIAN_POINT('Ctrl Pts',(38.327775614,12.870232221,5.52338273));
#168737=CARTESIAN_POINT('Ctrl Pts',(39.612362704,12.291625054,5.065558721));
#168738=CARTESIAN_POINT('Ctrl Pts',(39.096161745,12.852602028,5.140539372));
#168739=CARTESIAN_POINT('Ctrl Pts',(38.334045837,12.929709683,5.140305186));
#168740=CARTESIAN_POINT('Ctrl Pts',(39.616832291,12.327120707,4.813571576));
#168741=CARTESIAN_POINT('Ctrl Pts',(39.100604791,12.889321181,4.884922274));
#168742=CARTESIAN_POINT('Ctrl Pts',(38.337926232,12.96651201,4.884701294));
#168743=CARTESIAN_POINT('Ctrl Pts',(39.629202178,12.425400322,4.057017133));
#168744=CARTESIAN_POINT('Ctrl Pts',(39.112905272,12.991004201,4.117328691));
#168745=CARTESIAN_POINT('Ctrl Pts',(38.348668923,13.068413471,4.117224781));
#168746=CARTESIAN_POINT('Ctrl Pts',(39.636062814,12.479982592,3.551857239));
#168747=CARTESIAN_POINT('Ctrl Pts',(39.119729727,13.047470758,3.604789474));
#168748=CARTESIAN_POINT('Ctrl Pts',(38.354631783,13.125013103,3.604687756));
#168749=CARTESIAN_POINT('Ctrl Pts',(39.652544937,12.611040789,2.03393161));
#168750=CARTESIAN_POINT('Ctrl Pts',(39.13613297,13.183094783,2.064203406));
#168751=CARTESIAN_POINT('Ctrl Pts',(38.368964592,13.260927701,2.064336404));
#168752=CARTESIAN_POINT('Ctrl Pts',(39.658062289,12.654909258,1.018725573));
#168753=CARTESIAN_POINT('Ctrl Pts',(39.14162554,13.228470363,1.034037942));
#168754=CARTESIAN_POINT('Ctrl Pts',(38.37376987,13.306425053,1.034006735));
#168755=CARTESIAN_POINT('Ctrl Pts',(39.658062379,12.654909975,-1.018700666));
#168756=CARTESIAN_POINT('Ctrl Pts',(39.141625629,13.228471105,-1.034012664));
#168757=CARTESIAN_POINT('Ctrl Pts',(38.373769948,13.306425797,-1.033981454));
#168758=CARTESIAN_POINT('Ctrl Pts',(39.652545109,12.611042157,-2.033910583));
#168759=CARTESIAN_POINT('Ctrl Pts',(39.136133141,13.183096198,-2.064182064));
#168760=CARTESIAN_POINT('Ctrl Pts',(38.368964742,13.26092912,-2.064315063));
#168761=CARTESIAN_POINT('Ctrl Pts',(39.63606298,12.479983912,-3.55184454));
#168762=CARTESIAN_POINT('Ctrl Pts',(39.119729893,13.047472124,-3.604776588));
#168763=CARTESIAN_POINT('Ctrl Pts',(38.354631928,13.125014472,-3.604674871));
#168764=CARTESIAN_POINT('Ctrl Pts',(39.62920232,12.425401455,-4.057007807));
#168765=CARTESIAN_POINT('Ctrl Pts',(39.112905414,12.991005374,-4.117319229));
#168766=CARTESIAN_POINT('Ctrl Pts',(38.348669047,13.068414646,-4.117215321));
#168767=CARTESIAN_POINT('Ctrl Pts',(39.616832352,12.327121184,-4.813568203));
#168768=CARTESIAN_POINT('Ctrl Pts',(39.10060485,12.889321675,-4.884918852));
#168769=CARTESIAN_POINT('Ctrl Pts',(38.337926284,12.966512505,-4.884697873));
#168770=CARTESIAN_POINT('Ctrl Pts',(39.612362728,12.29162525,-5.065557481));
#168771=CARTESIAN_POINT('Ctrl Pts',(39.09616177,12.852602231,-5.140538114));
#168772=CARTESIAN_POINT('Ctrl Pts',(38.334045859,12.929709886,-5.140303928));
#168773=CARTESIAN_POINT('Ctrl Pts',(39.605137019,12.234256923,-5.443248896));
#168774=CARTESIAN_POINT('Ctrl Pts',(39.088980434,12.793254281,-5.523662297));
#168775=CARTESIAN_POINT('Ctrl Pts',(38.327775578,12.870231873,-5.523384943));
#168776=CARTESIAN_POINT('Ctrl Pts',(39.602642659,12.214455194,-5.569040712));
#168777=CARTESIAN_POINT('Ctrl Pts',(39.086501854,12.772770847,-5.651251005));
#168778=CARTESIAN_POINT('Ctrl Pts',(38.325611493,12.849702281,-5.650966557));
#168779=CARTESIAN_POINT('Ctrl Pts',(39.598773114,12.183737037,-5.757551029));
#168780=CARTESIAN_POINT('Ctrl Pts',(39.082657215,12.740994723,-5.842451499));
#168781=CARTESIAN_POINT('Ctrl Pts',(38.322255156,12.817855485,-5.842151243));
#168782=CARTESIAN_POINT('Ctrl Pts',(39.597461912,12.173328219,-5.820359327));
#168783=CARTESIAN_POINT('Ctrl Pts',(39.081354581,12.730227835,-5.906152889));
#168784=CARTESIAN_POINT('Ctrl Pts',(38.321117991,12.807064306,-5.905849292));
#168785=CARTESIAN_POINT('Ctrl Pts',(39.595962819,12.161427634,-5.890986684));
#168786=CARTESIAN_POINT('Ctrl Pts',(39.079865354,12.717917658,-5.97778472999999));
#168787=CARTESIAN_POINT('Ctrl Pts',(38.319818046,12.794726647,-5.977475704));
#168788=CARTESIAN_POINT('Ctrl Pts',(39.59579592,12.160102699,-5.898833724));
#168789=CARTESIAN_POINT('Ctrl Pts',(39.079699559,12.716547157,-5.985743153));
#168790=CARTESIAN_POINT('Ctrl Pts',(38.319673321,12.793353052,-5.985433723));
#168791=CARTESIAN_POINT('Ctrl Pts',(39.595461455,12.157447531,-5.914526915));
#168792=CARTESIAN_POINT('Ctrl Pts',(39.07936731,12.71380068,-6.001659054));
#168793=CARTESIAN_POINT('Ctrl Pts',(38.319383298,12.790600372,-6.001348821));
#168794=CARTESIAN_POINT('Ctrl Pts',(39.595293562,12.156117653,-5.922373124));
#168795=CARTESIAN_POINT('Ctrl Pts',(39.079205984,12.712477918,-6.00931156300001));
#168796=CARTESIAN_POINT('Ctrl Pts',(38.319247176,12.789313871,-6.008773556));
#168797=CARTESIAN_POINT('Ctrl Pts',(39.594778252,12.152131523,-5.945912251));
#168798=CARTESIAN_POINT('Ctrl Pts',(39.078708171,12.708490538,-6.03240212699999));
#168799=CARTESIAN_POINT('Ctrl Pts',(38.318823223,12.785418134,-6.031279663));
#168800=CARTESIAN_POINT('Ctrl Pts',(39.594422669,12.149475044,-5.961605075));
#168801=CARTESIAN_POINT('Ctrl Pts',(39.078364422,12.705833489,-6.04779593400001));
#168802=CARTESIAN_POINT('Ctrl Pts',(38.318528767,12.782822174,-6.046283705));
#168803=CARTESIAN_POINT('Ctrl Pts',(39.593963129,12.146155621,-5.981221196));
#168804=CARTESIAN_POINT('Ctrl Pts',(39.077919884,12.70251368,-6.067038345));
#168805=CARTESIAN_POINT('Ctrl Pts',(38.318145912,12.779578724,-6.065038719));
#168806=CARTESIAN_POINT('Ctrl Pts',(39.593870468,12.145491795,-5.985144425));
#168807=CARTESIAN_POINT('Ctrl Pts',(39.077830234,12.701849797,-6.070886809));
#168808=CARTESIAN_POINT('Ctrl Pts',(38.318068602,12.778930109,-6.06878972));
#168809=CARTESIAN_POINT('Ctrl Pts',(39.593683639,12.144164261,-5.992990892));
#168810=CARTESIAN_POINT('Ctrl Pts',(39.07764945,12.700522184,-6.078583744));
#168811=CARTESIAN_POINT('Ctrl Pts',(38.317912503,12.777633029,-6.076291718));
#168812=CARTESIAN_POINT('Ctrl Pts',(39.593577743,12.143490088,-5.997033475));
#168813=CARTESIAN_POINT('Ctrl Pts',(39.077549071,12.699847578,-6.082499696));
#168814=CARTESIAN_POINT('Ctrl Pts',(38.317833619,12.776984574,-6.080042715));
#168815=CARTESIAN_POINT('Ctrl Pts',(39.593338947,12.141540211,-6.008334875));
#168816=CARTESIAN_POINT('Ctrl Pts',(39.077309655,12.697899294,-6.093780331));
#168817=CARTESIAN_POINT('Ctrl Pts',(38.317595353,12.775039371,-6.091295702));
#168818=CARTESIAN_POINT('Ctrl Pts',(39.593186038,12.14024596,-6.015804605));
#168819=CARTESIAN_POINT('Ctrl Pts',(39.077154985,12.696606323,-6.101264269));
#168820=CARTESIAN_POINT('Ctrl Pts',(38.317436504,12.77374257,-6.098797693));
#168821=CARTESIAN_POINT('Ctrl Pts',(39.592717878,12.136354706,-6.0383106));
#168822=CARTESIAN_POINT('Ctrl Pts',(39.076683565,12.692718583,-6.123770813));
#168823=CARTESIAN_POINT('Ctrl Pts',(38.316959965,12.769852166,-6.121303667));
#168824=CARTESIAN_POINT('Ctrl Pts',(39.592405772,12.133760536,-6.053314596));
#168825=CARTESIAN_POINT('Ctrl Pts',(39.076369285,12.690126757,-6.13877517200001));
#168826=CARTESIAN_POINT('Ctrl Pts',(38.316642272,12.767258563,-6.136307649));
#168827=CARTESIAN_POINT('Ctrl Pts',(39.592093666,12.131166367,-6.068318593));
#168828=CARTESIAN_POINT('Ctrl Pts',(39.076055005,12.687534933,-6.153779523));
#168829=CARTESIAN_POINT('Ctrl Pts',(38.316324579,12.76466496,-6.151311631));
#168830=CARTESIAN_POINT('',(38.3194078266977,12.7908331451233,-5.99999998228311));
#168831=CARTESIAN_POINT('',(38.3194078268329,12.7908331478054,5.99999997429129));
#168832=CARTESIAN_POINT('Ctrl Pts',(38.3194078303931,12.7908331817173,-5.99999994684931));
#168833=CARTESIAN_POINT('Ctrl Pts',(38.3194475682192,12.7912087694162,-5.99783007957096));
#168834=CARTESIAN_POINT('Ctrl Pts',(38.3194876939326,12.7915891814127,-5.99563172340608));
#168835=CARTESIAN_POINT('Ctrl Pts',(38.319528521751,12.7919766905508,-5.99339127208654));
#168836=CARTESIAN_POINT('Ctrl Pts',(38.3196735650741,12.7933533404767,-5.98543193167468));
#168837=CARTESIAN_POINT('Ctrl Pts',(38.3198182890647,12.7947269337395,-5.97747391585236));
#168838=CARTESIAN_POINT('Ctrl Pts',(38.3199626941277,12.7960974767983,-5.96951721386296));
#168839=CARTESIAN_POINT('Ctrl Pts',(38.3211202440174,12.8070837395616,-5.9057363510682));
#168840=CARTESIAN_POINT('Ctrl Pts',(38.3222573068458,12.8178740050506,-5.84203994285522));
#168841=CARTESIAN_POINT('Ctrl Pts',(38.3233741257768,12.8284710643812,-5.77842301440819));
#168842=CARTESIAN_POINT('Ctrl Pts',(38.3256191940973,12.8497736422066,-5.65053804868484));
#168843=CARTESIAN_POINT('Ctrl Pts',(38.3277825389442,12.870296302613,-5.52296986150142));
#168844=CARTESIAN_POINT('Ctrl Pts',(38.3298658277331,12.8900578615479,-5.39569127138992));
#168845=CARTESIAN_POINT('Ctrl Pts',(38.3340708096828,12.9299452737301,-5.13878777493661));
#168846=CARTESIAN_POINT('Ctrl Pts',(38.3379460181326,12.966698589345,-4.88329627876836));
#168847=CARTESIAN_POINT('Ctrl Pts',(38.3415073042792,13.0004798752819,-4.62887035569616));
#168848=CARTESIAN_POINT('Ctrl Pts',(38.3455434470947,13.0387655083149,-4.34051965338579));
#168849=CARTESIAN_POINT('Ctrl Pts',(38.3491761736271,13.0732364223088,-4.05353783913861));
#168850=CARTESIAN_POINT('Ctrl Pts',(38.3524253407918,13.1040650384041,-3.76741605704691));
#168851=CARTESIAN_POINT('Ctrl Pts',(38.3549900677902,13.1283995770772,-3.54156610160221));
#168852=CARTESIAN_POINT('Ctrl Pts',(38.3573156958337,13.15046365334,-3.31625193559478));
#168853=CARTESIAN_POINT('Ctrl Pts',(38.3594095624069,13.1703193516511,-3.09122160167224));
#168854=CARTESIAN_POINT('Ctrl Pts',(38.3620840178367,13.1956806525291,-2.80379469198174));
#168855=CARTESIAN_POINT('Ctrl Pts',(38.3643798369784,13.2174459453909,-2.51684851920759));
#168856=CARTESIAN_POINT('Ctrl Pts',(38.3663038029257,13.2356826405251,-2.22985396662523));
#168857=CARTESIAN_POINT('Ctrl Pts',(38.3682262152592,13.2539046094208,-1.94309116383032));
#168858=CARTESIAN_POINT('Ctrl Pts',(38.3697773754982,13.2686036771062,-1.65628007016979));
#168859=CARTESIAN_POINT('Ctrl Pts',(38.3709586208108,13.2797955404709,-1.36888890983398));
#168860=CARTESIAN_POINT('Ctrl Pts',(38.3721352867201,13.2909440156785,-1.08261189576711));
#168861=CARTESIAN_POINT('Ctrl Pts',(38.3729449015694,13.2986124318983,-0.795759314868996));
#168862=CARTESIAN_POINT('Ctrl Pts',(38.3733833859369,13.3027651339286,-0.50780148111664));
#168863=CARTESIAN_POINT('Ctrl Pts',(38.373640502044,13.3052001730298,-0.338950313963452));
#168864=CARTESIAN_POINT('Ctrl Pts',(38.3737699088722,13.3064254242396,-0.169719044683042));
#168865=CARTESIAN_POINT('Ctrl Pts',(38.3737699090002,13.3064254250023,-1.99360232965105E-7));
#168866=CARTESIAN_POINT('Ctrl Pts',(38.3737699090002,13.3064254250023,4.08059336375396E-6));
#168867=CARTESIAN_POINT('Ctrl Pts',(38.3737699090002,13.3064254250015,8.36054677588611E-6));
#168868=CARTESIAN_POINT('Ctrl Pts',(38.373769909,13.306425425,1.26405000035384E-5));
#168869=CARTESIAN_POINT('Ctrl Pts',(38.3737698980774,13.306425320815,0.289600606570371));
#168870=CARTESIAN_POINT('Ctrl Pts',(38.3733934350627,13.302860883464,0.577769581499957));
#168871=CARTESIAN_POINT('Ctrl Pts',(38.3726478095811,13.2957981256462,0.865052432993628));
#168872=CARTESIAN_POINT('Ctrl Pts',(38.3719001282633,13.2887158944158,1.15312737982036));
#168873=CARTESIAN_POINT('Ctrl Pts',(38.3707812417038,13.2781159920207,1.44031129655557));
#168874=CARTESIAN_POINT('Ctrl Pts',(38.3692929967903,13.2640129059284,1.72713722866002));
#168875=CARTESIAN_POINT('Ctrl Pts',(38.3678024134377,13.2498876600381,2.014413842596));
#168876=CARTESIAN_POINT('Ctrl Pts',(38.3659413080516,13.2322482009507,2.30133133418495));
#168877=CARTESIAN_POINT('Ctrl Pts',(38.3637060723775,13.211057273523,2.58842120747477));
#168878=CARTESIAN_POINT('Ctrl Pts',(38.3624018526689,13.1986927494975,2.75593297154826));
#168879=CARTESIAN_POINT('Ctrl Pts',(38.3609701579466,13.185118156905,2.92350334827925));
#168880=CARTESIAN_POINT('Ctrl Pts',(38.3594094157851,13.1703179659798,3.09123730533891));
#168881=CARTESIAN_POINT('Ctrl Pts',(38.3567565033852,13.1451609535038,3.37634749558842));
#168882=CARTESIAN_POINT('Ctrl Pts',(38.3537317291153,13.1164605661736,3.66191318681091));
#168883=CARTESIAN_POINT('Ctrl Pts',(38.3503195989016,13.0840851791422,3.94844622381797));
#168884=CARTESIAN_POINT('Ctrl Pts',(38.3476268373177,13.0585353926433,4.17457040615839));
#168885=CARTESIAN_POINT('Ctrl Pts',(38.3446927302622,13.0306958640117,4.40129696805432));
#168886=CARTESIAN_POINT('Ctrl Pts',(38.3415072284282,13.0004791536001,4.62887578969621));
#168887=CARTESIAN_POINT('Ctrl Pts',(38.3379459614551,12.9666980483206,4.88330004794792));
#168888=CARTESIAN_POINT('Ctrl Pts',(38.3340707814642,12.9299450098084,5.13878942487707));
#168889=CARTESIAN_POINT('Ctrl Pts',(38.3298658446338,12.8900580258576,5.39569021538999));
#168890=CARTESIAN_POINT('Ctrl Pts',(38.3277825733939,12.8702966335071,5.52296775842875));
#168891=CARTESIAN_POINT('Ctrl Pts',(38.325619205431,12.849773747823,5.65053740685728));
#168892=CARTESIAN_POINT('Ctrl Pts',(38.3233741350629,12.8284711523523,5.77842248640831));
#168893=CARTESIAN_POINT('Ctrl Pts',(38.3222573136357,12.8178740702233,5.84203955564889));
#168894=CARTESIAN_POINT('Ctrl Pts',(38.3211202497904,12.8070837874715,5.90573607444173));
#168895=CARTESIAN_POINT('Ctrl Pts',(38.3199626977756,12.7960975110998,5.96951701541865));
#168896=CARTESIAN_POINT('Ctrl Pts',(38.3198182923721,12.7947269656274,5.97747373131824));
#168897=CARTESIAN_POINT('Ctrl Pts',(38.3196735683827,12.7933533693638,5.98543176114177));
#168898=CARTESIAN_POINT('Ctrl Pts',(38.3195285245693,12.7919767175187,5.99339111408667));
#168899=CARTESIAN_POINT('Ctrl Pts',(38.3194876958478,12.7915892005779,5.99563161092288));
#168900=CARTESIAN_POINT('Ctrl Pts',(38.3194475692977,12.791208780971,5.99783001162888));
#168901=CARTESIAN_POINT('Ctrl Pts',(38.3194078306652,12.7908331857559,5.99999992287387));
#168902=CARTESIAN_POINT('Ctrl Pts',(39.5935147999063,12.1429785426452,-6.));
#168903=CARTESIAN_POINT('Ctrl Pts',(39.4299502083,12.3246348464625,-6.));
#168904=CARTESIAN_POINT('Ctrl Pts',(39.2346482743456,12.4748234427719,-6.));
#168905=CARTESIAN_POINT('Ctrl Pts',(38.7990187662661,12.6966740224187,-6.));
#168906=CARTESIAN_POINT('Ctrl Pts',(38.5626404589734,12.7662707484543,-6.));
#168907=CARTESIAN_POINT('Ctrl Pts',(38.3194078294636,12.7908331725129,-6.));
#168908=CARTESIAN_POINT('Ctrl Pts',(38.3194078293165,12.7908331723995,6.));
#168909=CARTESIAN_POINT('Ctrl Pts',(38.5626163926011,12.7662731786021,6.));
#168910=CARTESIAN_POINT('Ctrl Pts',(38.7989722118466,12.6966877715691,6.));
#168911=CARTESIAN_POINT('Ctrl Pts',(39.234609763126,12.4748530096939,6.));
#168912=CARTESIAN_POINT('Ctrl Pts',(39.4299340103852,12.3246528308041,6.));
#168913=CARTESIAN_POINT('Ctrl Pts',(39.5935147874398,12.1429785566993,6.));
#168914=CARTESIAN_POINT('Ctrl Pts',(44.0515296615211,11.1342999421954,-6.00000101620338));
#168915=CARTESIAN_POINT('Ctrl Pts',(40.5316975951668,15.0434694841942,-6.00000101620338));
#168916=CARTESIAN_POINT('Ctrl Pts',(44.4394414973113,11.4835773287603,-2.01993501424746));
#168917=CARTESIAN_POINT('Ctrl Pts',(40.919609431951,15.392746870759,-2.01993501424746));
#168918=CARTESIAN_POINT('Ctrl Pts',(44.4394414972397,11.4835773286958,2.01993501645796));
#168919=CARTESIAN_POINT('Ctrl Pts',(40.9196094318794,15.3927468706946,2.01993501645796));
#168920=CARTESIAN_POINT('Ctrl Pts',(44.0515296613106,11.1342999420059,6.00000101836325));
#168921=CARTESIAN_POINT('Ctrl Pts',(40.5316975949563,15.0434694840047,6.00000101836325));
#168922=CARTESIAN_POINT('',(40.7532527139649,14.7974077937632,5.99999999957928));
#168923=CARTESIAN_POINT('',(40.7532527139641,14.7974077951072,-5.99999999785059));
#168924=CARTESIAN_POINT('Ctrl Pts',(40.7532527144433,14.7974077941939,5.99999999873785));
#168925=CARTESIAN_POINT('Ctrl Pts',(40.7532924812137,14.7976753308601,5.99840954433184));
#168926=CARTESIAN_POINT('Ctrl Pts',(40.7533491101781,14.7979581227393,5.99664529387617));
#168927=CARTESIAN_POINT('Ctrl Pts',(40.7534558041612,14.7985550657764,5.99299194501064));
#168928=CARTESIAN_POINT('Ctrl Pts',(40.7535129011557,14.7988755637752,5.99103053615936));
#168929=CARTESIAN_POINT('Ctrl Pts',(40.7536836381393,14.7998370887716,5.98514632460547));
#168930=CARTESIAN_POINT('Ctrl Pts',(40.7537967221284,14.8004781467692,5.98122353590287));
#168931=CARTESIAN_POINT('Ctrl Pts',(40.7548078250307,14.8062480357487,5.94591862257864));
#168932=CARTESIAN_POINT('Ctrl Pts',(40.755659241947,14.8113794517343,5.91453775695695));
#168933=CARTESIAN_POINT('Ctrl Pts',(40.7572675467857,14.8216475397135,5.85177854471206));
#168934=CARTESIAN_POINT('Ctrl Pts',(40.7580244347082,14.826784210707,5.82040019808882));
#168935=CARTESIAN_POINT('Ctrl Pts',(40.7588228446244,14.8325659217041,5.78510095276256));
#168936=CARTESIAN_POINT('Ctrl Pts',(40.7589108196152,14.8332083747038,5.78117883405955));
#168937=CARTESIAN_POINT('Ctrl Pts',(40.7590852955968,14.8344933637034,5.77333463465351));
#168938=CARTESIAN_POINT('Ctrl Pts',(40.7591716215836,14.8351360876644,5.76941258518122));
#168939=CARTESIAN_POINT('Ctrl Pts',(40.7594296415835,14.8370630319307,5.75764627249435));
#168940=CARTESIAN_POINT('Ctrl Pts',(40.7596013055834,14.8383450251078,5.74980168503647));
#168941=CARTESIAN_POINT('Ctrl Pts',(40.7601152485831,14.8421830976382,5.72626678466271));
#168942=CARTESIAN_POINT('Ctrl Pts',(40.7604564785829,14.8447312699902,5.710575334747));
#168943=CARTESIAN_POINT('Ctrl Pts',(40.7635149085818,14.8675700021467,5.56933862049449));
#168944=CARTESIAN_POINT('Ctrl Pts',(40.7661435385818,14.8871969748543,5.44369774616897));
#168945=CARTESIAN_POINT('Ctrl Pts',(40.7737551075852,14.9440621737053,5.06648121210239));
#168946=CARTESIAN_POINT('Ctrl Pts',(40.7784623225903,14.9792865425664,4.81461194334237));
#168947=CARTESIAN_POINT('Ctrl Pts',(40.7871545096106,15.0443529055857,4.31006932438241));
#168948=CARTESIAN_POINT('Ctrl Pts',(40.7911465216264,15.0741883397303,4.05738582923914));
#168949=CARTESIAN_POINT('Ctrl Pts',(40.7984000276565,15.1284728542493,3.55123173804321));
#168950=CARTESIAN_POINT('Ctrl Pts',(40.8016544526714,15.1528923416321,3.29806718191379));
#168951=CARTESIAN_POINT('Ctrl Pts',(40.8074403117045,15.196290473674,2.79154410222681));
#168952=CARTESIAN_POINT('Ctrl Pts',(40.8099783237223,15.2152618303147,2.5381852268234));
#168953=CARTESIAN_POINT('Ctrl Pts',(40.8143192897512,15.2477947438337,2.03125603914715));
#168954=CARTESIAN_POINT('Ctrl Pts',(40.8161208197628,15.2613578867193,1.77768580579081));
#168955=CARTESIAN_POINT('Ctrl Pts',(40.8204554687961,15.2939070022674,1.01662841704047));
#168956=CARTESIAN_POINT('Ctrl Pts',(40.8219101918083,15.3047673577721,0.508795305361927));
#168957=CARTESIAN_POINT('Ctrl Pts',(40.8219117688083,15.3047794997738,-0.507946056309606));
#168958=CARTESIAN_POINT('Ctrl Pts',(40.8204543377961,15.2938983532662,-1.0171588060745));
#168959=CARTESIAN_POINT('Ctrl Pts',(40.8161130907627,15.2612988407111,-1.7788985638649));
#168960=CARTESIAN_POINT('Ctrl Pts',(40.8143093397511,15.2477191338232,-2.03257819622708));
#168961=CARTESIAN_POINT('Ctrl Pts',(40.8099659147222,15.2151684783018,-2.53949227890163));
#168962=CARTESIAN_POINT('Ctrl Pts',(40.8074276987045,15.1961958996608,-2.79272657929782));
#168963=CARTESIAN_POINT('Ctrl Pts',(40.8016454686713,15.1528258396229,-3.29876580195453));
#168964=CARTESIAN_POINT('Ctrl Pts',(40.7983948646565,15.1284356312442,-3.55157138606291));
#168965=CARTESIAN_POINT('Ctrl Pts',(40.7911552316264,15.0742550937395,-4.05677442320306));
#168966=CARTESIAN_POINT('Ctrl Pts',(40.7871688846105,15.0444618076008,-4.30917160432941));
#168967=CARTESIAN_POINT('Ctrl Pts',(40.7784810945902,14.9794276565858,-4.81357265728204));
#168968=CARTESIAN_POINT('Ctrl Pts',(40.7737713965852,14.9441841657221,-5.06564351805385));
#168969=CARTESIAN_POINT('Ctrl Pts',(40.7661532925818,14.8872698388643,-5.44322870314176));
#168970=CARTESIAN_POINT('Ctrl Pts',(40.7635224655818,14.8676264361545,-5.56898398847384));
#168971=CARTESIAN_POINT('Ctrl Pts',(40.7604615915829,14.8447694529955,-5.71033991073328));
#168972=CARTESIAN_POINT('Ctrl Pts',(40.7601200905831,14.8422192556431,-5.72604447364975));
#168973=CARTESIAN_POINT('Ctrl Pts',(40.7596057415834,14.8383781521124,-5.74959884602463));
#168974=CARTESIAN_POINT('Ctrl Pts',(40.7594339415835,14.8370951489351,-5.75744989148289));
#168975=CARTESIAN_POINT('Ctrl Pts',(40.7591757195836,14.8351666916686,-5.76922584117032));
#168976=CARTESIAN_POINT('Ctrl Pts',(40.7590893545964,14.8345234327034,-5.7731510916674));
#168977=CARTESIAN_POINT('Ctrl Pts',(40.7589147826148,14.8332373917038,-5.78100169707296));
#168978=CARTESIAN_POINT('Ctrl Pts',(40.758826757624,14.8325944117041,-5.78492701777574));
#168979=CARTESIAN_POINT('Ctrl Pts',(40.7580278877079,14.826807971707,-5.8202550640998));
#168980=CARTESIAN_POINT('Ctrl Pts',(40.7572705177854,14.8216671167134,-5.85165891972112));
#168981=CARTESIAN_POINT('Ctrl Pts',(40.7556610989468,14.8113907007343,-5.91446896596217));
#168982=CARTESIAN_POINT('Ctrl Pts',(40.7548090520306,14.8062551397487,-5.94587515558194));
#168983=CARTESIAN_POINT('Ctrl Pts',(40.7537971561283,14.8004806117692,-5.98120845490401));
#168984=CARTESIAN_POINT('Ctrl Pts',(40.7536839831392,14.7998390387716,-5.98513439560637));
#168985=CARTESIAN_POINT('Ctrl Pts',(40.7535131111557,14.7988767407752,-5.9910233351599));
#168986=CARTESIAN_POINT('Ctrl Pts',(40.7534559681611,14.7985559857764,-5.99298631901107));
#168987=CARTESIAN_POINT('Ctrl Pts',(40.7533491890241,14.7979585651291,-5.99664258254315));
#168988=CARTESIAN_POINT('Ctrl Pts',(40.7532925113861,14.7976755455897,-5.99840827840234));
#168989=CARTESIAN_POINT('Ctrl Pts',(40.7532527155551,14.7974077965398,-5.99999999355178));
#168990=CARTESIAN_POINT('',(41.7359306993252,13.7060333274604,6.));
#168991=CARTESIAN_POINT('',(40.7532527143533,14.7974077953405,-6.));
#168992=CARTESIAN_POINT('Ctrl Pts',(9.758033795,14.612348562,6.));
#168993=CARTESIAN_POINT('Ctrl Pts',(10.542955148,14.611742111,6.));
#168994=CARTESIAN_POINT('Ctrl Pts',(11.32816556,14.591601296,6.));
#168995=CARTESIAN_POINT('Ctrl Pts',(12.113445943,14.550446495,6.));
#168996=CARTESIAN_POINT('Ctrl Pts',(9.763948215,14.780478266,5.009967665));
#168997=CARTESIAN_POINT('Ctrl Pts',(10.549810959,14.785748194,5.010318328));
#168998=CARTESIAN_POINT('Ctrl Pts',(11.33613133,14.768826884,5.01051229));
#168999=CARTESIAN_POINT('Ctrl Pts',(12.122730321,14.727602978,5.01051229));
#169000=CARTESIAN_POINT('Ctrl Pts',(9.771419064,15.033582243,3.014974832));
#169001=CARTESIAN_POINT('Ctrl Pts',(10.559011277,15.047679518,3.015501647));
#169002=CARTESIAN_POINT('Ctrl Pts',(11.347466763,15.035579093,3.015793043));
#169003=CARTESIAN_POINT('Ctrl Pts',(12.136702969,14.994216976,3.015793043));
#169004=CARTESIAN_POINT('Ctrl Pts',(9.774986833,15.160468498,0.));
#169005=CARTESIAN_POINT('Ctrl Pts',(10.563484757,15.178988749,0.));
#169006=CARTESIAN_POINT('Ctrl Pts',(11.353068133,15.169301939,0.));
#169007=CARTESIAN_POINT('Ctrl Pts',(12.143707233,15.127866299,0.));
#169008=CARTESIAN_POINT('Ctrl Pts',(9.771419064,15.033582243,-3.014974832));
#169009=CARTESIAN_POINT('Ctrl Pts',(10.559011277,15.047679518,-3.015501647));
#169010=CARTESIAN_POINT('Ctrl Pts',(11.347466763,15.035579093,-3.015793043));
#169011=CARTESIAN_POINT('Ctrl Pts',(12.136702969,14.994216976,-3.015793043));
#169012=CARTESIAN_POINT('Ctrl Pts',(9.763948215,14.780478266,-5.009967665));
#169013=CARTESIAN_POINT('Ctrl Pts',(10.549810959,14.785748194,-5.010318328));
#169014=CARTESIAN_POINT('Ctrl Pts',(11.33613133,14.768826884,-5.01051229));
#169015=CARTESIAN_POINT('Ctrl Pts',(12.122730321,14.727602978,-5.01051229));
#169016=CARTESIAN_POINT('Ctrl Pts',(9.758033795,14.612348562,-6.));
#169017=CARTESIAN_POINT('Ctrl Pts',(10.542955148,14.611742111,-6.));
#169018=CARTESIAN_POINT('Ctrl Pts',(11.32816556,14.591601296,-6.));
#169019=CARTESIAN_POINT('Ctrl Pts',(12.113445943,14.550446495,-6.));
#169020=CARTESIAN_POINT('Ctrl Pts',(9.7577972182,14.60562337384,-6.0396012934));
#169021=CARTESIAN_POINT('Ctrl Pts',(10.54268091556,14.60478186768,-6.03958726688));
#169022=CARTESIAN_POINT('Ctrl Pts',(11.3278469292,14.58451227248,-6.0395795084));
#169023=CARTESIAN_POINT('Ctrl Pts',(12.11307456788,14.54336023568,-6.0395795084));
#169024=CARTESIAN_POINT('Ctrl Pts',(9.7575606414,14.59889818568,-6.0792025868));
#169025=CARTESIAN_POINT('Ctrl Pts',(10.54240668312,14.59782162436,-6.07917453376));
#169026=CARTESIAN_POINT('Ctrl Pts',(11.3275282984,14.57742324896,-6.0791590168));
#169027=CARTESIAN_POINT('Ctrl Pts',(12.11270319276,14.53627397636,-6.0791590168));
#169028=CARTESIAN_POINT('Ctrl Pts',(9.7573240646,14.59217299752,-6.1188038802));
#169029=CARTESIAN_POINT('Ctrl Pts',(10.54213245068,14.59086138104,-6.11876180064));
#169030=CARTESIAN_POINT('Ctrl Pts',(11.3272096676,14.57033422544,-6.1187385252));
#169031=CARTESIAN_POINT('Ctrl Pts',(12.11233181764,14.52918771704,-6.1187385252));
#169032=CARTESIAN_POINT('',(9.79794790085819,14.6123008732764,-5.99999994854148));
#169033=CARTESIAN_POINT('',(12.1134459448026,14.5504464930284,-6.00000000166256));
#169034=CARTESIAN_POINT('Ctrl Pts',(9.79794877240227,14.6123008871254,-6.));
#169035=CARTESIAN_POINT('Ctrl Pts',(10.5695747870962,14.6110532742617,-6.));
#169036=CARTESIAN_POINT('Ctrl Pts',(11.3414765555483,14.5909036962831,-6.));
#169037=CARTESIAN_POINT('Ctrl Pts',(12.1134459457272,14.550446492489,-6.));
#169038=CARTESIAN_POINT('',(12.1134459448786,14.5504464944803,5.99999999961158));
#169039=CARTESIAN_POINT('Ctrl Pts',(12.1134459430031,14.5504464950543,5.99999999969675));
#169040=CARTESIAN_POINT('Ctrl Pts',(12.1320240607837,14.9049380944675,4.02002684265496));
#169041=CARTESIAN_POINT('Ctrl Pts',(12.141372478348,15.0833165249396,2.01154104533017));
#169042=CARTESIAN_POINT('Ctrl Pts',(12.1413724783187,15.0833165243943,-2.00789360499469));
#169043=CARTESIAN_POINT('Ctrl Pts',(12.1319903606165,14.9042950569859,-4.02361845730749));
#169044=CARTESIAN_POINT('Ctrl Pts',(12.1134459429818,14.5504464946533,-6.0000000019364));
#169045=CARTESIAN_POINT('',(9.79794823008933,14.612300878333,5.99999997397329));
#169046=CARTESIAN_POINT('Ctrl Pts',(12.1134459458125,14.5504464941161,6.));
#169047=CARTESIAN_POINT('Ctrl Pts',(11.3414766025522,14.5909036938197,6.));
#169048=CARTESIAN_POINT('Ctrl Pts',(10.5695748810957,14.611053271808,6.));
#169049=CARTESIAN_POINT('Ctrl Pts',(9.79794891334272,14.6123008817038,6.));
#169050=CARTESIAN_POINT('Ctrl Pts',(9.79794788859268,14.6123008832888,5.99999992191988));
#169051=CARTESIAN_POINT('Ctrl Pts',(9.7979500800566,14.6125894414009,5.99830368000664));
#169052=CARTESIAN_POINT('Ctrl Pts',(9.79794640227073,14.6129084799895,5.99642789963154));
#169053=CARTESIAN_POINT('Ctrl Pts',(9.79794507046349,14.6132150280573,5.9946244480845));
#169054=CARTESIAN_POINT('Ctrl Pts',(9.79794343836482,14.6135906955563,5.99241436032496));
#169055=CARTESIAN_POINT('Ctrl Pts',(9.797941820851,14.6139659648138,5.99020535120621));
#169056=CARTESIAN_POINT('Ctrl Pts',(9.79794021861651,14.6143408380001,5.98799741265409));
#169057=CARTESIAN_POINT('Ctrl Pts',(9.7978525587376,14.6348505313159,5.86719884872445));
#169058=CARTESIAN_POINT('Ctrl Pts',(9.79781066749895,14.654180848725,5.74959401446796));
#169059=CARTESIAN_POINT('Ctrl Pts',(9.79779333553231,14.6726038633972,5.63405188307487));
#169060=CARTESIAN_POINT('Ctrl Pts',(9.79777555264829,14.691506180708,5.51550374808145));
#169061=CARTESIAN_POINT('Ctrl Pts',(9.79778348353759,14.709453307596,5.39912677717061));
#169062=CARTESIAN_POINT('Ctrl Pts',(9.7977873569103,14.7266861962401,5.28368727150186));
#169063=CARTESIAN_POINT('Ctrl Pts',(9.7977889900763,14.7339522586037,5.23501344410497));
#169064=CARTESIAN_POINT('Ctrl Pts',(9.79778983197078,14.7410907159002,5.1865061574113));
#169065=CARTESIAN_POINT('Ctrl Pts',(9.79778738507617,14.7481169257174,5.13807247881662));
#169066=CARTESIAN_POINT('Ctrl Pts',(9.79778153561427,14.7649135406528,5.0222885966929));
#169067=CARTESIAN_POINT('Ctrl Pts',(9.79775791998702,14.7810703528341,4.90694343321932));
#169068=CARTESIAN_POINT('Ctrl Pts',(9.79767818984793,14.7967638304198,4.79074603437952));
#169069=CARTESIAN_POINT('Ctrl Pts',(9.79761438680368,14.8093223391131,4.69776052269151));
#169070=CARTESIAN_POINT('Ctrl Pts',(9.7975145594496,14.8215831841756,4.60422918585069));
#169071=CARTESIAN_POINT('Ctrl Pts',(9.79735797733189,14.8336128666801,4.50948853860347));
#169072=CARTESIAN_POINT('Ctrl Pts',(9.79676530749574,14.879145715919,4.15089124342981));
#169073=CARTESIAN_POINT('Ctrl Pts',(9.7959450021984,14.9192348565256,3.79157351780402));
#169074=CARTESIAN_POINT('Ctrl Pts',(9.7950926075,14.953868669,3.431707731));
#169075=CARTESIAN_POINT('Ctrl Pts',(9.79479733986455,14.9658657449263,3.30705101956353));
#169076=CARTESIAN_POINT('Ctrl Pts',(9.79449812915568,14.9772078235421,3.18232915770469));
#169077=CARTESIAN_POINT('Ctrl Pts',(9.79420022074329,14.9878944220546,3.0575485461174));
#169078=CARTESIAN_POINT('Ctrl Pts',(9.79416286827072,14.9892343334541,3.04190325321103));
#169079=CARTESIAN_POINT('Ctrl Pts',(9.79412148215503,14.9907073476449,3.02455621728992));
#169080=CARTESIAN_POINT('Ctrl Pts',(9.79407243535764,14.9918830187537,3.01060967259255));
#169081=CARTESIAN_POINT('Ctrl Pts',(9.79309389504961,15.0153390164952,2.73235998313183));
#169082=CARTESIAN_POINT('Ctrl Pts',(9.79230021516519,15.0364330462044,2.44325467676033));
#169083=CARTESIAN_POINT('Ctrl Pts',(9.79166768385037,15.0543911195385,2.14337439862685));
#169084=CARTESIAN_POINT('Ctrl Pts',(9.79137351457374,15.0627428221633,2.00391005524037));
#169085=CARTESIAN_POINT('Ctrl Pts',(9.79111458808493,15.0704156336338,1.86211527147687));
#169086=CARTESIAN_POINT('Ctrl Pts',(9.79089069072951,15.0773285435866,1.71799844027648));
#169087=CARTESIAN_POINT('Ctrl Pts',(9.79082384392684,15.0793924622362,1.67497091385613));
#169088=CARTESIAN_POINT('Ctrl Pts',(9.79076001954289,15.0813886874519,1.63173316511455));
#169089=CARTESIAN_POINT('Ctrl Pts',(9.79069913107378,15.0833149579498,1.58828679378095));
#169090=CARTESIAN_POINT('Ctrl Pts',(9.79040718463865,15.0925509892244,1.3799712717242));
#169091=CARTESIAN_POINT('Ctrl Pts',(9.79018370715181,15.1001791149284,1.166892959045));
#169092=CARTESIAN_POINT('Ctrl Pts',(9.7900219600675,15.1059476883998,0.949060540766124));
#169093=CARTESIAN_POINT('Ctrl Pts',(9.78999962212445,15.1067443523165,0.918976980526512));
#169094=CARTESIAN_POINT('Ctrl Pts',(9.78997846820551,15.1075055117168,0.88880281833857));
#169095=CARTESIAN_POINT('Ctrl Pts',(9.78995848711913,15.1082304671688,0.858538147994024));
#169096=CARTESIAN_POINT('Ctrl Pts',(9.78994886882902,15.1085794387775,0.843969651862457));
#169097=CARTESIAN_POINT('Ctrl Pts',(9.78993952235631,15.1089200241747,0.829380448721482));
#169098=CARTESIAN_POINT('Ctrl Pts',(9.78993044359277,15.1092521483247,0.814770493349579));
#169099=CARTESIAN_POINT('Ctrl Pts',(9.78984819129214,15.1122611456734,0.682406384993954));
#169100=CARTESIAN_POINT('Ctrl Pts',(9.78978793063445,15.1145760536446,0.54832419543522));
#169101=CARTESIAN_POINT('Ctrl Pts',(9.78974823694479,15.116138994976,0.412531798708623));
#169102=CARTESIAN_POINT('Ctrl Pts',(9.78972839009996,15.1169204656416,0.344635600345324));
#169103=CARTESIAN_POINT('Ctrl Pts',(9.78971368534993,15.1175139282023,0.276311850322579));
#169104=CARTESIAN_POINT('Ctrl Pts',(9.7897039406203,15.1179120533349,0.207561686381522));
#169105=CARTESIAN_POINT('Ctrl Pts',(9.78969906825549,15.1181111159013,0.173186604410992));
#169106=CARTESIAN_POINT('Ctrl Pts',(9.78969543591472,15.1182613431959,0.138704918937019));
#169107=CARTESIAN_POINT('Ctrl Pts',(9.78969302078614,15.1183618136691,0.104116776811358));
#169108=CARTESIAN_POINT('Ctrl Pts',(9.78969181322185,15.1184120489057,0.086822705748525));
#169109=CARTESIAN_POINT('Ctrl Pts',(9.78969090996175,15.1184498448821,0.0695020205216681));
#169110=CARTESIAN_POINT('Ctrl Pts',(9.78969030814099,15.1184750860797,0.0521547400165017));
#169111=CARTESIAN_POINT('Ctrl Pts',(9.7896900072306,15.1184877066784,0.0434810997639184));
#169112=CARTESIAN_POINT('Ctrl Pts',(9.78968978168012,15.1184971885791,0.0348008106916684));
#169113=CARTESIAN_POINT('Ctrl Pts',(9.78968963113053,15.1185035173221,0.0261138751957106));
#169114=CARTESIAN_POINT('Ctrl Pts',(9.78968948058094,15.1185098460651,0.0174269396997527));
#169115=CARTESIAN_POINT('Ctrl Pts',(9.78968940485914,15.1185130231695,0.00707187686119539));
#169116=CARTESIAN_POINT('Ctrl Pts',(9.78968940412529,15.1185130296052,3.31318431472039E-5));
#169117=CARTESIAN_POINT('Ctrl Pts',(9.78968940408767,15.118513029935,-0.000327672777262212));
#169118=CARTESIAN_POINT('Ctrl Pts',(9.78968940427655,15.1185130248193,-0.000688494058382274));
#169119=CARTESIAN_POINT('Ctrl Pts',(9.78968940469201,15.1185130142563,-0.00104933199997106));
#169120=CARTESIAN_POINT('Ctrl Pts',(9.78968974774507,15.1185042923071,-0.2989969357337));
#169121=CARTESIAN_POINT('Ctrl Pts',(9.78985105637987,15.1147891306134,-0.608259091370153));
#169122=CARTESIAN_POINT('Ctrl Pts',(9.79018146417964,15.1064875059098,-0.928699572294281));
#169123=CARTESIAN_POINT('Ctrl Pts',(9.7903502600005,15.1022464451443,-1.0924033772587));
#169124=CARTESIAN_POINT('Ctrl Pts',(9.7905630345956,15.0968075421677,-1.25902473626515));
#169125=CARTESIAN_POINT('Ctrl Pts',(9.79081980750076,15.0900484174663,-1.42854638429469));
#169126=CARTESIAN_POINT('Ctrl Pts',(9.79096469902433,15.0862343862492,-1.5242038674947));
#169127=CARTESIAN_POINT('Ctrl Pts',(9.79112358631072,15.0819999450171,-1.62078414142528));
#169128=CARTESIAN_POINT('Ctrl Pts',(9.79129635633333,15.077322754,-1.71828248833332));
#169129=CARTESIAN_POINT('Ctrl Pts',(9.79166409101511,15.0673675237795,-1.92580415807717));
#169130=CARTESIAN_POINT('Ctrl Pts',(9.79209231393233,15.0554054190377,-2.13748477179792));
#169131=CARTESIAN_POINT('Ctrl Pts',(9.79256487626909,15.0412094777158,-2.35327968127705));
#169132=CARTESIAN_POINT('Ctrl Pts',(9.79272641854607,15.0363566900376,-2.42704772905783));
#169133=CARTESIAN_POINT('Ctrl Pts',(9.79289309842739,15.031242840242,-2.50129592942567));
#169134=CARTESIAN_POINT('Ctrl Pts',(9.7930641305,15.0258588495,-2.57602044850002));
#169135=CARTESIAN_POINT('Ctrl Pts',(9.79327367392242,15.019262543736,-2.66757071288625));
#169136=CARTESIAN_POINT('Ctrl Pts',(9.79348974652061,15.0122597715775,-2.75984220914934));
#169137=CARTESIAN_POINT('Ctrl Pts',(9.793710077335,15.0048341883609,-2.8528254936469));
#169138=CARTESIAN_POINT('Ctrl Pts',(9.79375208732067,15.0034183689469,-2.87055440941397));
#169139=CARTESIAN_POINT('Ctrl Pts',(9.79379425160075,15.0019871723335,-2.88830926034111));
#169140=CARTESIAN_POINT('Ctrl Pts',(9.79383655358928,15.0005404799128,-2.90609001439213));
#169141=CARTESIAN_POINT('Ctrl Pts',(9.79387734925027,14.9991453026262,-2.92323761524699));
#169142=CARTESIAN_POINT('Ctrl Pts',(9.79391827298526,14.9977357134172,-2.94040930776202));
#169143=CARTESIAN_POINT('Ctrl Pts',(9.79395926806275,14.9963116044282,-2.95760506283209));
#169144=CARTESIAN_POINT('Ctrl Pts',(9.79400026314025,14.9948874954392,-2.97480081790216));
#169145=CARTESIAN_POINT('Ctrl Pts',(9.79404510637553,14.9933149759388,-2.99360933560658));
#169146=CARTESIAN_POINT('Ctrl Pts',(9.79408255626668,14.9919956115203,-3.00926448860491));
#169147=CARTESIAN_POINT('Ctrl Pts',(9.79442367992096,14.9799777818834,-3.15186418208799));
#169148=CARTESIAN_POINT('Ctrl Pts',(9.7946910709083,14.9672240920578,-3.29298618374894));
#169149=CARTESIAN_POINT('Ctrl Pts',(9.79490867824321,14.9537238032509,-3.43318591187827));
#169150=CARTESIAN_POINT('Ctrl Pts',(9.79516006594659,14.9381277912901,-3.59514960525305));
#169151=CARTESIAN_POINT('Ctrl Pts',(9.79534662111358,14.9215405704387,-3.75586458296582));
#169152=CARTESIAN_POINT('Ctrl Pts',(9.79550146245736,14.9038907416998,-3.91628227532854));
#169153=CARTESIAN_POINT('Ctrl Pts',(9.79565616962082,14.8862562077119,-4.07656095508648));
#169154=CARTESIAN_POINT('Ctrl Pts',(9.79577935812821,14.867560891691,-4.23654284284504));
#169155=CARTESIAN_POINT('Ctrl Pts',(9.79590288664792,14.8476821414815,-4.39716987604912));
#169156=CARTESIAN_POINT('Ctrl Pts',(9.79602515559278,14.8280060875706,-4.55615905452083));
#169157=CARTESIAN_POINT('Ctrl Pts',(9.79614789577125,14.8071706176418,-4.71578026901489));
#169158=CARTESIAN_POINT('Ctrl Pts',(9.79629879439229,14.7850065463336,-4.87694037663787));
#169159=CARTESIAN_POINT('Ctrl Pts',(9.79638035986249,14.7730261658288,-4.96405250439962));
#169160=CARTESIAN_POINT('Ctrl Pts',(9.79647008533354,14.7606567345884,-5.05161414583504));
#169161=CARTESIAN_POINT('Ctrl Pts',(9.79657172109791,14.7478652436572,-5.13976773370651));
#169162=CARTESIAN_POINT('Ctrl Pts',(9.79675360190473,14.7249744167373,-5.29752170728039));
#169163=CARTESIAN_POINT('Ctrl Pts',(9.79697275033504,14.7007341922703,-5.45717140418589));
#169164=CARTESIAN_POINT('Ctrl Pts',(9.79724085837546,14.6749163120254,-5.61952745024738));
#169165=CARTESIAN_POINT('Ctrl Pts',(9.79744138183986,14.6556065935176,-5.74095684405289));
#169166=CARTESIAN_POINT('Ctrl Pts',(9.79766917912186,14.6354134211619,-5.86390001075217));
#169167=CARTESIAN_POINT('Ctrl Pts',(9.79792567385572,14.6142226062327,-5.98869386966598));
#169168=CARTESIAN_POINT('Ctrl Pts',(9.79793345018516,14.6135801495424,-5.99247733197415));
#169169=CARTESIAN_POINT('Ctrl Pts',(9.79794791329567,14.6129018735453,-5.99646672715746));
#169170=CARTESIAN_POINT('Ctrl Pts',(9.7979474653736,14.6123008794813,-5.99999984562444));
#169171=CARTESIAN_POINT('Ctrl Pts',(12.1123317552017,14.5291866595917,6.11874443277285));
#169172=CARTESIAN_POINT('Ctrl Pts',(20.8902575146672,14.2345980190016,6.11876772761178));
#169173=CARTESIAN_POINT('Ctrl Pts',(29.5936684411877,13.65102255426,6.11879102245071));
#169174=CARTESIAN_POINT('Ctrl Pts',(38.3179610775993,12.7701867243602,6.11881431716964));
#169175=CARTESIAN_POINT('Ctrl Pts',(38.3699704723074,12.7649356698709,6.11881445601655));
#169176=CARTESIAN_POINT('Ctrl Pts',(38.4219798682553,12.7596846155016,6.11881459486345));
#169177=CARTESIAN_POINT('Ctrl Pts',(38.4739892629633,12.7544335598922,6.11881473383037));
#169178=CARTESIAN_POINT('Ctrl Pts',(12.1127031487985,14.5362732714729,6.0791629551819));
#169179=CARTESIAN_POINT('Ctrl Pts',(20.8907773155674,14.2416052037713,6.07917848507452));
#169180=CARTESIAN_POINT('Ctrl Pts',(29.5943366493513,13.6579503119182,6.07919401496715));
#169181=CARTESIAN_POINT('Ctrl Pts',(38.3187776930662,12.7770350549068,6.07920954477976));
#169182=CARTESIAN_POINT('Ctrl Pts',(38.3707879725382,12.7717835269139,6.07920963734436));
#169183=CARTESIAN_POINT('Ctrl Pts',(38.4227982531702,12.766531999001,6.07920972990897));
#169184=CARTESIAN_POINT('Ctrl Pts',(38.4748085326422,12.7612804699281,6.07920982255358));
#169185=CARTESIAN_POINT('Ctrl Pts',(12.1130745423953,14.5433598833541,6.03958147759095));
#169186=CARTESIAN_POINT('Ctrl Pts',(20.8912971164676,14.248612388541,6.03958924253726));
#169187=CARTESIAN_POINT('Ctrl Pts',(29.5950048575148,13.6648780695763,6.03959700748357));
#169188=CARTESIAN_POINT('Ctrl Pts',(38.3195943085331,12.7838833854534,6.03960477238988));
#169189=CARTESIAN_POINT('Ctrl Pts',(38.3716054727691,12.778631383957,6.03960481867218));
#169190=CARTESIAN_POINT('Ctrl Pts',(38.4236166380851,12.7733793825005,6.03960486495448));
#169191=CARTESIAN_POINT('Ctrl Pts',(38.4756278023211,12.7681273799641,6.03960491127679));
#169192=CARTESIAN_POINT('Ctrl Pts',(12.1134459359922,14.5504464952354,6.));
#169193=CARTESIAN_POINT('Ctrl Pts',(20.8918169173678,14.2556195733107,6.));
#169194=CARTESIAN_POINT('Ctrl Pts',(29.5956730656783,13.6718058272345,6.));
#169195=CARTESIAN_POINT('Ctrl Pts',(38.320410924,12.790731716,6.));
#169196=CARTESIAN_POINT('Ctrl Pts',(38.372422973,12.785479241,6.));
#169197=CARTESIAN_POINT('Ctrl Pts',(38.424435023,12.780226766,6.));
#169198=CARTESIAN_POINT('Ctrl Pts',(38.476447072,12.77497429,6.));
#169199=CARTESIAN_POINT('Ctrl Pts',(12.1227303139892,14.7276029782369,5.01051229000016));
#169200=CARTESIAN_POINT('Ctrl Pts',(20.9048112933658,14.4307904773118,5.0103181760001));
#169201=CARTESIAN_POINT('Ctrl Pts',(29.6123774386773,13.844991152235,5.01012406200005));
#169202=CARTESIAN_POINT('Ctrl Pts',(38.340825295,12.961931462,5.009929949));
#169203=CARTESIAN_POINT('Ctrl Pts',(38.392859462,12.95666715,5.009928792));
#169204=CARTESIAN_POINT('Ctrl Pts',(38.444893628,12.951402837,5.009927635));
#169205=CARTESIAN_POINT('Ctrl Pts',(38.496927795,12.946138525,5.009926477));
#169206=CARTESIAN_POINT('Ctrl Pts',(12.1367029619847,14.9942169762393,3.01579304300023));
#169207=CARTESIAN_POINT('Ctrl Pts',(20.9243654493628,14.6944005693134,3.01550099000015));
#169208=CARTESIAN_POINT('Ctrl Pts',(29.6375131046759,14.1055973392358,3.01520893700008));
#169209=CARTESIAN_POINT('Ctrl Pts',(38.37154247,13.219533743,3.014916884));
#169210=CARTESIAN_POINT('Ctrl Pts',(38.42360991,13.214251523,3.014915143));
#169211=CARTESIAN_POINT('Ctrl Pts',(38.47567735,13.208969303,3.014913402));
#169212=CARTESIAN_POINT('Ctrl Pts',(38.527744791,13.203687083,3.014911661));
#169213=CARTESIAN_POINT('Ctrl Pts',(12.1437072259825,15.1278662992405,0.));
#169214=CARTESIAN_POINT('Ctrl Pts',(20.9341668943613,14.8265379783142,0.));
#169215=CARTESIAN_POINT('Ctrl Pts',(29.6501117306751,14.2362228332362,0.));
#169216=CARTESIAN_POINT('Ctrl Pts',(38.386938276,13.348647322,0.));
#169217=CARTESIAN_POINT('Ctrl Pts',(38.439022392,13.343356089,0.));
#169218=CARTESIAN_POINT('Ctrl Pts',(38.491106507,13.338064856,0.));
#169219=CARTESIAN_POINT('Ctrl Pts',(38.543190623,13.332773623,0.));
#169220=CARTESIAN_POINT('Ctrl Pts',(12.1367029619847,14.9942169762393,-3.01579304300023));
#169221=CARTESIAN_POINT('Ctrl Pts',(20.9243654493628,14.6944005693134,-3.01550099000015));
#169222=CARTESIAN_POINT('Ctrl Pts',(29.6375131046759,14.1055973392358,-3.01520893700008));
#169223=CARTESIAN_POINT('Ctrl Pts',(38.37154247,13.219533743,-3.014916884));
#169224=CARTESIAN_POINT('Ctrl Pts',(38.42360991,13.214251523,-3.014915143));
#169225=CARTESIAN_POINT('Ctrl Pts',(38.47567735,13.208969303,-3.014913402));
#169226=CARTESIAN_POINT('Ctrl Pts',(38.527744791,13.203687083,-3.014911661));
#169227=CARTESIAN_POINT('Ctrl Pts',(12.1227303139892,14.7276029782369,-5.01051229000016));
#169228=CARTESIAN_POINT('Ctrl Pts',(20.9048112933658,14.4307904773118,-5.0103181760001));
#169229=CARTESIAN_POINT('Ctrl Pts',(29.6123774386773,13.844991152235,-5.01012406200005));
#169230=CARTESIAN_POINT('Ctrl Pts',(38.340825295,12.961931462,-5.009929949));
#169231=CARTESIAN_POINT('Ctrl Pts',(38.392859462,12.95666715,-5.009928792));
#169232=CARTESIAN_POINT('Ctrl Pts',(38.444893628,12.951402837,-5.009927635));
#169233=CARTESIAN_POINT('Ctrl Pts',(38.496927795,12.946138525,-5.009926477));
#169234=CARTESIAN_POINT('Ctrl Pts',(12.1134459359922,14.5504464952354,-6.));
#169235=CARTESIAN_POINT('Ctrl Pts',(20.8918169173678,14.2556195733107,-6.));
#169236=CARTESIAN_POINT('Ctrl Pts',(29.5956730656783,13.6718058272345,-6.));
#169237=CARTESIAN_POINT('Ctrl Pts',(38.320410924,12.790731716,-6.));
#169238=CARTESIAN_POINT('Ctrl Pts',(38.372422973,12.785479241,-6.));
#169239=CARTESIAN_POINT('Ctrl Pts',(38.424435023,12.780226766,-6.));
#169240=CARTESIAN_POINT('Ctrl Pts',(38.476447072,12.77497429,-6.));
#169241=CARTESIAN_POINT('Ctrl Pts',(12.1134440882973,14.5504112391184,-6.00019691909556));
#169242=CARTESIAN_POINT('Ctrl Pts',(20.891814331342,14.2555847123461,-6.00019695772641));
#169243=CARTESIAN_POINT('Ctrl Pts',(29.5956697413217,13.6717713614223,-6.00019699635726));
#169244=CARTESIAN_POINT('Ctrl Pts',(38.3204068613124,12.7906976453402,-6.00019703498792));
#169245=CARTESIAN_POINT('Ctrl Pts',(38.3724189059106,12.7854451726959,-6.00019703521817));
#169246=CARTESIAN_POINT('Ctrl Pts',(38.4244309515093,12.7801927000518,-6.00019703544843));
#169247=CARTESIAN_POINT('Ctrl Pts',(38.4764429961076,12.7749402264073,-6.00019703567888));
#169248=CARTESIAN_POINT('Ctrl Pts',(12.1134422406025,14.5503759830015,-6.00039383819112));
#169249=CARTESIAN_POINT('Ctrl Pts',(20.8918117453161,14.2555498513816,-6.00039391545282));
#169250=CARTESIAN_POINT('Ctrl Pts',(29.5956664169651,13.6717368956101,-6.00039399271453));
#169251=CARTESIAN_POINT('Ctrl Pts',(38.3204027986247,12.7906635746804,-6.00039406997583));
#169252=CARTESIAN_POINT('Ctrl Pts',(38.3724148388213,12.7854111043918,-6.00039407043634));
#169253=CARTESIAN_POINT('Ctrl Pts',(38.4244268800187,12.7801586341036,-6.00039407089686));
#169254=CARTESIAN_POINT('Ctrl Pts',(38.4764389202152,12.7749061628146,-6.00039407135776));
#169255=CARTESIAN_POINT('Ctrl Pts',(12.1134403929077,14.5503407268846,-6.00059075728668));
#169256=CARTESIAN_POINT('Ctrl Pts',(20.8918091592903,14.255514990417,-6.00059087317923));
#169257=CARTESIAN_POINT('Ctrl Pts',(29.5956630926085,13.6717024297979,-6.00059098907179));
#169258=CARTESIAN_POINT('Ctrl Pts',(38.3203987359371,12.7906295040206,-6.00059110496375));
#169259=CARTESIAN_POINT('Ctrl Pts',(38.3724107717319,12.7853770360877,-6.00059110565452));
#169260=CARTESIAN_POINT('Ctrl Pts',(38.4244228085279,12.7801245681554,-6.00059110634528));
#169261=CARTESIAN_POINT('Ctrl Pts',(38.4764348443227,12.7748720992219,-6.00059110703665));
#169262=CARTESIAN_POINT('Ctrl Pts',(12.1134459458125,14.5504464941161,6.));
#169263=CARTESIAN_POINT('Ctrl Pts',(20.8914804963054,14.2556308720613,6.));
#169264=CARTESIAN_POINT('Ctrl Pts',(29.5950059279722,13.6718505751845,6.));
#169265=CARTESIAN_POINT('Ctrl Pts',(38.3194078205169,12.7908330852606,6.));
#169266=CARTESIAN_POINT('Ctrl Pts',(12.1134459457272,14.550446492489,-6.));
#169267=CARTESIAN_POINT('Ctrl Pts',(20.8914804963505,14.2556308720598,-6.));
#169268=CARTESIAN_POINT('Ctrl Pts',(29.5950059280615,13.6718505751785,-6.));
#169269=CARTESIAN_POINT('Ctrl Pts',(38.3194078202364,12.7908330811398,-6.));
#169270=CARTESIAN_POINT('Ctrl Pts',(40.751918853,14.786422254,6.063606532));
#169271=CARTESIAN_POINT('Ctrl Pts',(39.491202843,16.145755581,6.271940406));
#169272=CARTESIAN_POINT('Ctrl Pts',(37.638148242,16.362045517,6.270436567));
#169273=CARTESIAN_POINT('Ctrl Pts',(40.752211793,14.788834877,6.049637389));
#169274=CARTESIAN_POINT('Ctrl Pts',(39.491495482,16.148168529,6.257971313));
#169275=CARTESIAN_POINT('Ctrl Pts',(37.638440405,16.364458231,6.256467424));
#169276=CARTESIAN_POINT('Ctrl Pts',(40.752504733,14.791247501,6.035668246));
#169277=CARTESIAN_POINT('Ctrl Pts',(39.491788121,16.150581477,6.244002221));
#169278=CARTESIAN_POINT('Ctrl Pts',(37.638732567,16.366870945,6.242498282));
#169279=CARTESIAN_POINT('Ctrl Pts',(40.752944143,14.794866436,6.014714532));
#169280=CARTESIAN_POINT('Ctrl Pts',(39.492227079,16.154200899,6.223048583));
#169281=CARTESIAN_POINT('Ctrl Pts',(37.639170812,16.370490016,6.221544569));
#169282=CARTESIAN_POINT('Ctrl Pts',(40.7530804,14.796063549,6.007834764));
#169283=CARTESIAN_POINT('Ctrl Pts',(39.492365431,16.15539798,6.216122968));
#169284=CARTESIAN_POINT('Ctrl Pts',(37.639316897,16.371696373,6.214559998));
#169285=CARTESIAN_POINT('Ctrl Pts',(40.753276253,14.797582938,5.998973045));
#169286=CARTESIAN_POINT('Ctrl Pts',(39.492558289,16.156917814,6.20731862));
#169287=CARTESIAN_POINT('Ctrl Pts',(37.639499494,16.37320432,6.205829284));
#169288=CARTESIAN_POINT('Ctrl Pts',(40.753343234,14.797911941,5.996914444));
#169289=CARTESIAN_POINT('Ctrl Pts',(39.492618548,16.157247449,6.205396776));
#169290=CARTESIAN_POINT('Ctrl Pts',(37.639535929,16.373505919,6.204083141));
#169291=CARTESIAN_POINT('Ctrl Pts',(40.753457798,14.798552916,5.992991615));
#169292=CARTESIAN_POINT('Ctrl Pts',(39.492723845,16.157889349,6.201662396));
#169293=CARTESIAN_POINT('Ctrl Pts',(37.639608365,16.374109168,6.200590857));
#169294=CARTESIAN_POINT('Ctrl Pts',(40.753514895,14.798873414,5.991030206));
#169295=CARTESIAN_POINT('Ctrl Pts',(39.492776315,16.158210319,6.19979521));
#169296=CARTESIAN_POINT('Ctrl Pts',(37.639644408,16.374410813,6.198844716));
#169297=CARTESIAN_POINT('Ctrl Pts',(40.753685632,14.799834939,5.985145994));
#169298=CARTESIAN_POINT('Ctrl Pts',(39.492933191,16.159173296,6.194193656));
#169299=CARTESIAN_POINT('Ctrl Pts',(37.639752006,16.375315808,6.193606291));
#169300=CARTESIAN_POINT('Ctrl Pts',(40.753798716,14.800475997,5.981223205));
#169301=CARTESIAN_POINT('Ctrl Pts',(39.493037062,16.159815364,6.190459303));
#169302=CARTESIAN_POINT('Ctrl Pts',(37.639823034,16.375919221,6.19011401));
#169303=CARTESIAN_POINT('Ctrl Pts',(40.754809819,14.806245886,5.945918289));
#169304=CARTESIAN_POINT('Ctrl Pts',(39.493965505,16.165594803,6.15684982700001));
#169305=CARTESIAN_POINT('Ctrl Pts',(37.640455947,16.381350669,6.158683494));
#169306=CARTESIAN_POINT('Ctrl Pts',(40.755661236,14.811377302,5.914537421));
#169307=CARTESIAN_POINT('Ctrl Pts',(39.494745181,16.17073739,6.12697600200001));
#169308=CARTESIAN_POINT('Ctrl Pts',(37.640973468,16.386183859,6.130745355));
#169309=CARTESIAN_POINT('Ctrl Pts',(40.757269541,14.82164539,5.851778204));
#169310=CARTESIAN_POINT('Ctrl Pts',(39.496213487,16.181033294,6.067230117));
#169311=CARTESIAN_POINT('Ctrl Pts',(37.641918511,16.395860698,6.074869273));
#169312=CARTESIAN_POINT('Ctrl Pts',(40.758026429,14.826782061,5.820399855));
#169313=CARTESIAN_POINT('Ctrl Pts',(39.496902116,16.186186614,6.037358037));
#169314=CARTESIAN_POINT('Ctrl Pts',(37.642346032,16.400704345,6.04693133));
#169315=CARTESIAN_POINT('Ctrl Pts',(40.758824839,14.832563772,5.785100607));
#169316=CARTESIAN_POINT('Ctrl Pts',(39.497625681,16.19199005,6.003753372));
#169317=CARTESIAN_POINT('Ctrl Pts',(37.642776444,16.406159322,6.015501255));
#169318=CARTESIAN_POINT('Ctrl Pts',(40.758912814,14.833206225,5.781178488));
#169319=CARTESIAN_POINT('Ctrl Pts',(39.497705368,16.192634969,6.000019484));
#169320=CARTESIAN_POINT('Ctrl Pts',(37.642823566,16.406765512,6.012009026));
#169321=CARTESIAN_POINT('Ctrl Pts',(40.75908729,14.834491214,5.773334288));
#169322=CARTESIAN_POINT('Ctrl Pts',(39.497863322,16.193924974,5.992551733));
#169323=CARTESIAN_POINT('Ctrl Pts',(37.642916405,16.407978056,6.00502457));
#169324=CARTESIAN_POINT('Ctrl Pts',(40.759173616,14.835133938,5.769412238));
#169325=CARTESIAN_POINT('Ctrl Pts',(39.497938817,16.194545702,5.988963843));
#169326=CARTESIAN_POINT('Ctrl Pts',(37.642956809,16.408540394,6.001788326));
#169327=CARTESIAN_POINT('Ctrl Pts',(40.759431636,14.837060882,5.757645926));
#169328=CARTESIAN_POINT('Ctrl Pts',(39.498189989,16.196648331,5.976764337));
#169329=CARTESIAN_POINT('Ctrl Pts',(37.643127719,16.410661213,5.98956156));
#169330=CARTESIAN_POINT('Ctrl Pts',(40.7596033,14.838342875,5.749801339));
#169331=CARTESIAN_POINT('Ctrl Pts',(39.4983571,16.198047194,5.968630971));
#169332=CARTESIAN_POINT('Ctrl Pts',(37.643241434,16.41207217,5.981410069));
#169333=CARTESIAN_POINT('Ctrl Pts',(40.760117243,14.842180947,5.72626644));
#169334=CARTESIAN_POINT('Ctrl Pts',(39.498857423,16.202235148,5.944229649));
#169335=CARTESIAN_POINT('Ctrl Pts',(37.643581901,16.416296281,5.956954638));
#169336=CARTESIAN_POINT('Ctrl Pts',(40.760458473,14.844729119,5.710574991));
#169337=CARTESIAN_POINT('Ctrl Pts',(39.49918962,16.205015569,5.92796064400001));
#169338=CARTESIAN_POINT('Ctrl Pts',(37.643807975,16.419100674,5.940649741));
#169339=CARTESIAN_POINT('Ctrl Pts',(40.763516903,14.867567848,5.569338285));
#169340=CARTESIAN_POINT('Ctrl Pts',(39.502167359,16.229936868,5.781518502));
#169341=CARTESIAN_POINT('Ctrl Pts',(37.645834449,16.444235233,5.793893783));
#169342=CARTESIAN_POINT('Ctrl Pts',(40.766145533,14.887194818,5.443697418));
#169343=CARTESIAN_POINT('Ctrl Pts',(39.504727246,16.251350544,5.65125599));
#169344=CARTESIAN_POINT('Ctrl Pts',(37.647577316,16.465830819,5.663359465));
#169345=CARTESIAN_POINT('Ctrl Pts',(40.773757102,14.944060009,5.066480906));
#169346=CARTESIAN_POINT('Ctrl Pts',(39.512141767,16.313397558,5.260113506));
#169347=CARTESIAN_POINT('Ctrl Pts',(37.652624545,16.528398406,5.271436973));
#169348=CARTESIAN_POINT('Ctrl Pts',(40.778464317,14.979284373,4.814611652));
#169349=CARTESIAN_POINT('Ctrl Pts',(39.516728629,16.351831306,4.998925481));
#169350=CARTESIAN_POINT('Ctrl Pts',(37.655745497,16.567154219,5.009728965));
#169351=CARTESIAN_POINT('Ctrl Pts',(40.787156504,15.044350727,4.310069063));
#169352=CARTESIAN_POINT('Ctrl Pts',(39.525205623,16.422852721,4.475459016));
#169353=CARTESIAN_POINT('Ctrl Pts',(37.661519285,16.638782663,4.485122415));
#169354=CARTESIAN_POINT('Ctrl Pts',(40.791148516,15.074186157,4.057385583));
#169355=CARTESIAN_POINT('Ctrl Pts',(39.529103262,16.455424856,4.213206507));
#169356=CARTESIAN_POINT('Ctrl Pts',(37.664181346,16.67163853,4.222264054));
#169357=CARTESIAN_POINT('Ctrl Pts',(40.798402022,15.128470664,3.551231522));
#169358=CARTESIAN_POINT('Ctrl Pts',(39.536185784,16.514676164,3.687964953));
#169359=CARTESIAN_POINT('Ctrl Pts',(37.669014595,16.731388256,3.69595042));
#169360=CARTESIAN_POINT('Ctrl Pts',(40.801656447,15.152890148,3.298066981));
#169361=CARTESIAN_POINT('Ctrl Pts',(39.539364042,16.541330737,3.425233638));
#169362=CARTESIAN_POINT('Ctrl Pts',(37.671180991,16.758266063,3.432694695));
#169363=CARTESIAN_POINT('Ctrl Pts',(40.807442306,15.196288274,2.791543932));
#169364=CARTESIAN_POINT('Ctrl Pts',(39.545018929,16.588720601,2.899300501));
#169365=CARTESIAN_POINT('Ctrl Pts',(37.675040966,16.806064026,2.905577901));
#169366=CARTESIAN_POINT('Ctrl Pts',(40.809980318,15.215259628,2.538185072));
#169367=CARTESIAN_POINT('Ctrl Pts',(39.547501902,16.609436799,2.636196155));
#169368=CARTESIAN_POINT('Ctrl Pts',(37.676741572,16.826959804,2.641874102));
#169369=CARTESIAN_POINT('Ctrl Pts',(40.814321284,15.247792537,2.031255915));
#169370=CARTESIAN_POINT('Ctrl Pts',(39.551747285,16.644956426,2.109854465));
#169371=CARTESIAN_POINT('Ctrl Pts',(37.679642934,16.862777999,2.114451962));
#169372=CARTESIAN_POINT('Ctrl Pts',(40.816122814,15.261355678,1.777685697));
#169373=CARTESIAN_POINT('Ctrl Pts',(39.553508565,16.659766031,1.846564618));
#169374=CARTESIAN_POINT('Ctrl Pts',(37.680842993,16.87771189,1.850627796));
#169375=CARTESIAN_POINT('Ctrl Pts',(40.820457463,15.293904789,1.016628355));
#169376=CARTESIAN_POINT('Ctrl Pts',(39.557750402,16.695321176,1.055911698));
#169377=CARTESIAN_POINT('Ctrl Pts',(37.68374148,16.913574407,1.058156218));
#169378=CARTESIAN_POINT('Ctrl Pts',(40.821912186,15.304765143,0.508795274));
#169379=CARTESIAN_POINT('Ctrl Pts',(39.559174912,16.707176419,0.528653896));
#169380=CARTESIAN_POINT('Ctrl Pts',(37.684718817,16.925528918,0.529898357));
#169381=CARTESIAN_POINT('Ctrl Pts',(40.821913763,15.304777285,-0.507946025));
#169382=CARTESIAN_POINT('Ctrl Pts',(39.559176451,16.707189689,-0.527771518));
#169383=CARTESIAN_POINT('Ctrl Pts',(37.684719848,16.925542301,-0.529013884));
#169384=CARTESIAN_POINT('Ctrl Pts',(40.820456332,15.29389614,-1.017158744));
#169385=CARTESIAN_POINT('Ctrl Pts',(39.557749268,16.695311724,-1.056463633));
#169386=CARTESIAN_POINT('Ctrl Pts',(37.683740661,16.913564823,-1.058710206));
#169387=CARTESIAN_POINT('Ctrl Pts',(40.816115085,15.261296632,-1.778898455));
#169388=CARTESIAN_POINT('Ctrl Pts',(39.553501,16.659701558,-1.847824273));
#169389=CARTESIAN_POINT('Ctrl Pts',(37.680837852,16.877646856,-1.851890285));
#169390=CARTESIAN_POINT('Ctrl Pts',(40.814311334,15.247716927,-2.032578072));
#169391=CARTESIAN_POINT('Ctrl Pts',(39.551737559,16.644873885,-2.111227207));
#169392=CARTESIAN_POINT('Ctrl Pts',(37.679636331,16.862694772,-2.115827428));
#169393=CARTESIAN_POINT('Ctrl Pts',(40.809967909,15.215166276,-2.539492124));
#169394=CARTESIAN_POINT('Ctrl Pts',(39.547489787,16.609334903,-2.637552708));
#169395=CARTESIAN_POINT('Ctrl Pts',(37.676733338,16.826857089,-2.643233108));
#169396=CARTESIAN_POINT('Ctrl Pts',(40.807429693,15.1961937,-2.792726409));
#169397=CARTESIAN_POINT('Ctrl Pts',(39.545006622,16.58861734,-2.900527902));
#169398=CARTESIAN_POINT('Ctrl Pts',(37.675032605,16.805959925,-2.906807665));
#169399=CARTESIAN_POINT('Ctrl Pts',(40.801647463,15.152823646,-3.298765601));
#169400=CARTESIAN_POINT('Ctrl Pts',(39.539355283,16.541258183,-3.425958027));
#169401=CARTESIAN_POINT('Ctrl Pts',(37.671175018,16.758192963,-3.433419989));
#169402=CARTESIAN_POINT('Ctrl Pts',(40.798396859,15.128433441,-3.55157117));
#169403=CARTESIAN_POINT('Ctrl Pts',(39.536180742,16.514635557,-3.688317055));
#169404=CARTESIAN_POINT('Ctrl Pts',(37.669011107,16.731347348,-3.696302854));
#169405=CARTESIAN_POINT('Ctrl Pts',(40.791157226,15.074252911,-4.056774177));
#169406=CARTESIAN_POINT('Ctrl Pts',(39.52911174,16.455497695,-4.212572296));
#169407=CARTESIAN_POINT('Ctrl Pts',(37.664187034,16.671711959,-4.22162859));
#169408=CARTESIAN_POINT('Ctrl Pts',(40.787170879,15.044459629,-4.309171343));
#169409=CARTESIAN_POINT('Ctrl Pts',(39.525219617,16.422971569,-4.474527811));
#169410=CARTESIAN_POINT('Ctrl Pts',(37.661528724,16.63890248,-4.484189389));
#169411=CARTESIAN_POINT('Ctrl Pts',(40.778483089,14.979425487,-4.813572366));
#169412=CARTESIAN_POINT('Ctrl Pts',(39.516746897,16.351985238,-4.997848097));
#169413=CARTESIAN_POINT('Ctrl Pts',(37.655757861,16.567309376,-5.008649756));
#169414=CARTESIAN_POINT('Ctrl Pts',(40.773773391,14.944182001,-5.065643212));
#169415=CARTESIAN_POINT('Ctrl Pts',(39.512157622,16.313530625,-5.259245174));
#169416=CARTESIAN_POINT('Ctrl Pts',(37.652635302,16.528532533,-5.270567207));
#169417=CARTESIAN_POINT('Ctrl Pts',(40.766155287,14.887267682,-5.443228375));
#169418=CARTESIAN_POINT('Ctrl Pts',(39.504736741,16.251430029,-5.650769785));
#169419=CARTESIAN_POINT('Ctrl Pts',(37.647583772,16.46591096,-5.662872346));
#169420=CARTESIAN_POINT('Ctrl Pts',(40.76352446,14.867624282,-5.568983653));
#169421=CARTESIAN_POINT('Ctrl Pts',(39.502174716,16.229998438,-5.781150848));
#169422=CARTESIAN_POINT('Ctrl Pts',(37.645839455,16.444297322,-5.793525384));
#169423=CARTESIAN_POINT('Ctrl Pts',(40.760463586,14.844767302,-5.710339567));
#169424=CARTESIAN_POINT('Ctrl Pts',(39.499194598,16.20505723,-5.927716562));
#169425=CARTESIAN_POINT('Ctrl Pts',(37.643811362,16.419142693,-5.940405128));
#169426=CARTESIAN_POINT('Ctrl Pts',(40.760122085,14.842217105,-5.726044129));
#169427=CARTESIAN_POINT('Ctrl Pts',(39.498862136,16.2022746,-5.94399916));
#169428=CARTESIAN_POINT('Ctrl Pts',(37.643585108,16.416336073,-5.956723643));
#169429=CARTESIAN_POINT('Ctrl Pts',(40.759607736,14.838376002,-5.7495985));
#169430=CARTESIAN_POINT('Ctrl Pts',(39.498361418,16.19808334,-5.968420666));
#169431=CARTESIAN_POINT('Ctrl Pts',(37.643244372,16.412108628,-5.981199297));
#169432=CARTESIAN_POINT('Ctrl Pts',(40.759435936,14.837092999,-5.757449545));
#169433=CARTESIAN_POINT('Ctrl Pts',(39.498194175,16.196683375,-5.976560726));
#169434=CARTESIAN_POINT('Ctrl Pts',(37.643130568,16.410696561,-5.989357496));
#169435=CARTESIAN_POINT('Ctrl Pts',(40.759177714,14.835164542,-5.769225494));
#169436=CARTESIAN_POINT('Ctrl Pts',(39.497942806,16.194579097,-5.988770223));
#169437=CARTESIAN_POINT('Ctrl Pts',(37.642959524,16.408574077,-6.001594272));
#169438=CARTESIAN_POINT('Ctrl Pts',(40.759091349,14.834521283,-5.773150745));
#169439=CARTESIAN_POINT('Ctrl Pts',(39.497866996,16.193955161,-5.992376998));
#169440=CARTESIAN_POINT('Ctrl Pts',(37.642918555,16.40800643,-6.004861143));
#169441=CARTESIAN_POINT('Ctrl Pts',(40.758916777,14.833235242,-5.781001351));
#169442=CARTESIAN_POINT('Ctrl Pts',(39.497708956,16.192664097,-5.999850847));
#169443=CARTESIAN_POINT('Ctrl Pts',(37.642825683,16.406792891,-6.011851303));
#169444=CARTESIAN_POINT('Ctrl Pts',(40.758828752,14.832592262,-5.784926672));
#169445=CARTESIAN_POINT('Ctrl Pts',(39.497629226,16.19201865,-6.003587784));
#169446=CARTESIAN_POINT('Ctrl Pts',(37.642778544,16.406186204,-6.015346383));
#169447=CARTESIAN_POINT('Ctrl Pts',(40.758029882,14.826805822,-5.820254721));
#169448=CARTESIAN_POINT('Ctrl Pts',(39.496905256,16.186210456,-6.037219868));
#169449=CARTESIAN_POINT('Ctrl Pts',(37.642347965,16.400726754,-6.046802108));
#169450=CARTESIAN_POINT('Ctrl Pts',(40.757272512,14.821664967,-5.851658579));
#169451=CARTESIAN_POINT('Ctrl Pts',(39.496216195,16.18105293,-6.067116234));
#169452=CARTESIAN_POINT('Ctrl Pts',(37.641920222,16.395879153,-6.074762766));
#169453=CARTESIAN_POINT('Ctrl Pts',(40.755663093,14.811388551,-5.91446863));
#169454=CARTESIAN_POINT('Ctrl Pts',(39.494746881,16.170748665,-6.126910513));
#169455=CARTESIAN_POINT('Ctrl Pts',(37.640974594,16.386194455,-6.13068411));
#169456=CARTESIAN_POINT('Ctrl Pts',(40.754811046,14.80625299,-5.945874822));
#169457=CARTESIAN_POINT('Ctrl Pts',(39.49396663,16.165601921,-6.156808447));
#169458=CARTESIAN_POINT('Ctrl Pts',(37.640456709,16.381357358,-6.158644796));
#169459=CARTESIAN_POINT('Ctrl Pts',(40.75379915,14.800478462,-5.981208124));
#169460=CARTESIAN_POINT('Ctrl Pts',(39.493037461,16.159817832,-6.190444947));
#169461=CARTESIAN_POINT('Ctrl Pts',(37.639823306,16.375921541,-6.190100585));
#169462=CARTESIAN_POINT('Ctrl Pts',(40.753685977,14.799836889,-5.985134065));
#169463=CARTESIAN_POINT('Ctrl Pts',(39.492933508,16.159175248,-6.1941823));
#169464=CARTESIAN_POINT('Ctrl Pts',(37.639752223,16.375317643,-6.193595672));
#169465=CARTESIAN_POINT('Ctrl Pts',(40.753515105,14.798874591,-5.991023005));
#169466=CARTESIAN_POINT('Ctrl Pts',(39.492776507,16.158211498,-6.199788354));
#169467=CARTESIAN_POINT('Ctrl Pts',(37.63964454,16.37441192,-6.198838304));
#169468=CARTESIAN_POINT('Ctrl Pts',(40.753457962,14.798553836,-5.992985989));
#169469=CARTESIAN_POINT('Ctrl Pts',(39.492723996,16.157890269,-6.20165704));
#169470=CARTESIAN_POINT('Ctrl Pts',(37.639608469,16.374110033,-6.200585848));
#169471=CARTESIAN_POINT('Ctrl Pts',(40.753343306,14.797912345,-5.996911967));
#169472=CARTESIAN_POINT('Ctrl Pts',(39.492618615,16.157247854,-6.205394418));
#169473=CARTESIAN_POINT('Ctrl Pts',(37.639535975,16.3735063,-6.204080937));
#169474=CARTESIAN_POINT('Ctrl Pts',(40.753276266,14.797583073,-5.998972286));
#169475=CARTESIAN_POINT('Ctrl Pts',(39.492558303,16.156917949,-6.20731784200001));
#169476=CARTESIAN_POINT('Ctrl Pts',(37.639499511,16.373204459,-6.205828481));
#169477=CARTESIAN_POINT('Ctrl Pts',(40.753080287,14.796062493,-6.007840791));
#169478=CARTESIAN_POINT('Ctrl Pts',(39.492365314,16.155396924,-6.21612907300001));
#169479=CARTESIAN_POINT('Ctrl Pts',(37.639316767,16.371695301,-6.214566202));
#169480=CARTESIAN_POINT('Ctrl Pts',(40.752943895,14.794864397,-6.014726342));
#169481=CARTESIAN_POINT('Ctrl Pts',(39.492226832,16.154198859,-6.22306039200001));
#169482=CARTESIAN_POINT('Ctrl Pts',(37.639170565,16.370487977,-6.221556379));
#169483=CARTESIAN_POINT('Ctrl Pts',(40.752504133,14.791242557,-6.035696874));
#169484=CARTESIAN_POINT('Ctrl Pts',(39.491787521,16.150576532,-6.244030848));
#169485=CARTESIAN_POINT('Ctrl Pts',(37.638731969,16.366866001,-6.242526909));
#169486=CARTESIAN_POINT('Ctrl Pts',(40.752210958,14.788827997,-6.049677228));
#169487=CARTESIAN_POINT('Ctrl Pts',(39.491494647,16.148161647,-6.258011152));
#169488=CARTESIAN_POINT('Ctrl Pts',(37.638439571,16.36445135,-6.256507263));
#169489=CARTESIAN_POINT('Ctrl Pts',(40.751917783,14.786413437,-6.063657583));
#169490=CARTESIAN_POINT('Ctrl Pts',(39.491201774,16.145746763,-6.271991456));
#169491=CARTESIAN_POINT('Ctrl Pts',(37.638147174,16.3620367,-6.270487617));
#169492=CARTESIAN_POINT('',(37.642982287708,16.4088504732111,6.0000000045992));
#169493=CARTESIAN_POINT('Ctrl Pts',(40.7532527124878,14.7974077924331,6.));
#169494=CARTESIAN_POINT('Ctrl Pts',(40.7041458477828,14.8519463637135,6.));
#169495=CARTESIAN_POINT('Ctrl Pts',(40.6538706170833,14.9053759733606,6.));
#169496=CARTESIAN_POINT('Ctrl Pts',(40.5506448722851,15.010356926483,6.));
#169497=CARTESIAN_POINT('Ctrl Pts',(40.4977017931235,15.0618690951414,6.));
#169498=CARTESIAN_POINT('Ctrl Pts',(40.3346211356183,15.2136538826667,6.));
#169499=CARTESIAN_POINT('Ctrl Pts',(40.2211264418376,15.310195291988,5.99999999999999));
#169500=CARTESIAN_POINT('Ctrl Pts',(39.8658746237043,15.5859305264852,5.99999999999999));
#169501=CARTESIAN_POINT('Ctrl Pts',(39.6120785669462,15.7484508164354,6.));
#169502=CARTESIAN_POINT('Ctrl Pts',(38.8138839016999,16.1625756328312,6.));
#169503=CARTESIAN_POINT('Ctrl Pts',(38.2373926026142,16.3395581228118,6.));
#169504=CARTESIAN_POINT('Ctrl Pts',(37.6429823003743,16.408850490623,6.));
#169505=CARTESIAN_POINT('',(37.6429823613304,16.4088504659907,-6.0000000042585));
#169506=CARTESIAN_POINT('Ctrl Pts',(40.7532527120421,14.7974077933766,-6.));
#169507=CARTESIAN_POINT('Ctrl Pts',(40.7041462463511,14.8519459198948,-6.));
#169508=CARTESIAN_POINT('Ctrl Pts',(40.6538706921651,14.9053758982138,-6.));
#169509=CARTESIAN_POINT('Ctrl Pts',(40.5506448319582,15.010356966506,-6.));
#169510=CARTESIAN_POINT('Ctrl Pts',(40.4977017441792,15.0618691421542,-6.));
#169511=CARTESIAN_POINT('Ctrl Pts',(40.3346210695018,15.2136539406401,-6.));
#169512=CARTESIAN_POINT('Ctrl Pts',(40.2211263668839,15.3101953538551,-5.99999999999999));
#169513=CARTESIAN_POINT('Ctrl Pts',(39.8658745654662,15.5859305633178,-5.99999999999999));
#169514=CARTESIAN_POINT('Ctrl Pts',(39.6120785407188,15.7484508290523,-6.));
#169515=CARTESIAN_POINT('Ctrl Pts',(38.8138839072929,16.1625756319594,-6.));
#169516=CARTESIAN_POINT('Ctrl Pts',(38.2373926217034,16.3395581146185,-6.));
#169517=CARTESIAN_POINT('Ctrl Pts',(37.6429823707101,16.4088504849673,-6.));
#169518=CARTESIAN_POINT('Ctrl Pts',(37.6429823002787,16.4088504893088,6.0000000075678));
#169519=CARTESIAN_POINT('Ctrl Pts',(37.6429925922719,16.4089782150111,5.99926381250339));
#169520=CARTESIAN_POINT('Ctrl Pts',(37.6430033422842,16.4091100012393,5.99850405484267));
#169521=CARTESIAN_POINT('Ctrl Pts',(37.6430147153378,16.4092472256471,5.9977127308646));
#169522=CARTESIAN_POINT('Ctrl Pts',(37.643131982462,16.4106621413092,5.98955341935717));
#169523=CARTESIAN_POINT('Ctrl Pts',(37.6432488657212,16.4120727214878,5.98140193700194));
#169524=CARTESIAN_POINT('Ctrl Pts',(37.6433653672416,16.413479002002,5.97325818682279));
#169525=CARTESIAN_POINT('Ctrl Pts',(37.6435990613265,16.4162999045681,5.95692238073991));
#169526=CARTESIAN_POINT('Ctrl Pts',(37.6438312194001,16.4191035056322,5.94061768806421));
#169527=CARTESIAN_POINT('Ctrl Pts',(37.6440618602537,16.4218900884576,5.924343327567));
#169528=CARTESIAN_POINT('Ctrl Pts',(37.6459383777535,16.4445620104253,5.79193347133972));
#169529=CARTESIAN_POINT('Ctrl Pts',(37.6477143696341,16.4661094409072,5.66153131418037));
#169530=CARTESIAN_POINT('Ctrl Pts',(37.6494005148935,16.4866704133275,5.53271773759048));
#169531=CARTESIAN_POINT('Ctrl Pts',(37.6515766957273,16.5132069135807,5.36646774523038));
#169532=CARTESIAN_POINT('Ctrl Pts',(37.6536026100879,16.5381029580661,5.20286396472447));
#169533=CARTESIAN_POINT('Ctrl Pts',(37.6555042291047,16.5615958150815,5.04100789616993));
#169534=CARTESIAN_POINT('Ctrl Pts',(37.6566607841939,16.5758840521591,4.94256785209843));
#169535=CARTESIAN_POINT('Ctrl Pts',(37.6577712692573,16.5896522020657,4.84477428699897));
#169536=CARTESIAN_POINT('Ctrl Pts',(37.6588407221678,16.6029443150722,4.74742454727631));
#169537=CARTESIAN_POINT('Ctrl Pts',(37.6606256646561,16.6251291696188,4.5849455031368));
#169538=CARTESIAN_POINT('Ctrl Pts',(37.6623000107574,16.6459842024763,4.42371918013501));
#169539=CARTESIAN_POINT('Ctrl Pts',(37.6638766613543,16.6656642734245,4.26289497760677));
#169540=CARTESIAN_POINT('Ctrl Pts',(37.6648702582042,16.678066549832,4.16154441753981));
#169541=CARTESIAN_POINT('Ctrl Pts',(37.665824986514,16.6900011746096,4.06035325873642));
#169542=CARTESIAN_POINT('Ctrl Pts',(37.6667432984757,16.7014965325222,3.95910657464045));
#169543=CARTESIAN_POINT('Ctrl Pts',(37.6682023425559,16.7197607331537,3.79824253146168));
#169544=CARTESIAN_POINT('Ctrl Pts',(37.6695678772653,16.7369126495672,3.63731299534655));
#169545=CARTESIAN_POINT('Ctrl Pts',(37.6708542262411,16.7530337280781,3.47534718421044));
#169546=CARTESIAN_POINT('Ctrl Pts',(37.6716610042114,16.7631446165251,3.37376475921804));
#169547=CARTESIAN_POINT('Ctrl Pts',(37.67243655048,16.7728489995321,3.27177465177766));
#169548=CARTESIAN_POINT('Ctrl Pts',(37.6731835960051,16.7821566076102,3.16913603168301));
#169549=CARTESIAN_POINT('Ctrl Pts',(37.6736139439681,16.7875184095921,3.11000935251626));
#169550=CARTESIAN_POINT('Ctrl Pts',(37.6740351776649,16.7927471664175,3.05067533514802));
#169551=CARTESIAN_POINT('Ctrl Pts',(37.6744473409751,16.79784346694,2.99109183013576));
#169552=CARTESIAN_POINT('Ctrl Pts',(37.6758619748775,16.8153350760109,2.7865883138774));
#169553=CARTESIAN_POINT('Ctrl Pts',(37.6771323103164,16.8310053965011,2.5821957216556));
#169554=CARTESIAN_POINT('Ctrl Pts',(37.6782497341041,16.8448622153274,2.37816287453634));
#169555=CARTESIAN_POINT('Ctrl Pts',(37.6796980785756,16.8628226768462,2.11370649784581));
#169556=CARTESIAN_POINT('Ctrl Pts',(37.6808888047079,16.8777467837798,1.84974709873201));
#169557=CARTESIAN_POINT('Ctrl Pts',(37.6818433082319,16.8896620864771,1.5864705405855));
#169558=CARTESIAN_POINT('Ctrl Pts',(37.6828847653763,16.9026628526441,1.29920994329351));
#169559=CARTESIAN_POINT('Ctrl Pts',(37.6836391356913,16.912070715238,1.01317287593597));
#169560=CARTESIAN_POINT('Ctrl Pts',(37.6841128849961,16.9179769777172,0.728685437826341));
#169561=CARTESIAN_POINT('Ctrl Pts',(37.6845191434982,16.9230418280994,0.484726366463135));
#169562=CARTESIAN_POINT('Ctrl Pts',(37.6847191100984,16.9255325562844,0.24190685609632));
#169563=CARTESIAN_POINT('Ctrl Pts',(37.6847193418195,16.9255356084144,0.000442236499989826));
#169564=CARTESIAN_POINT('Ctrl Pts',(37.6847193420007,16.9255356108004,0.000253469149640141));
#169565=CARTESIAN_POINT('Ctrl Pts',(37.6847193420595,16.9255356116628,6.47027496648115E-5));
#169566=CARTESIAN_POINT('Ctrl Pts',(37.684719341996,16.9255356110016,-0.000124062699716917));
#169567=CARTESIAN_POINT('Ctrl Pts',(37.6847192386803,16.9255345349064,-0.30734925937092));
#169568=CARTESIAN_POINT('Ctrl Pts',(37.6843947361347,16.9214935383538,-0.616974244090195));
#169569=CARTESIAN_POINT('Ctrl Pts',(37.6837342985532,16.9132579103563,-0.928286699200675));
#169570=CARTESIAN_POINT('Ctrl Pts',(37.683269727296,16.9074647269285,-1.1472730541378));
#169571=CARTESIAN_POINT('Ctrl Pts',(37.6826390212237,16.8995969890998,-1.36709393472077));
#169572=CARTESIAN_POINT('Ctrl Pts',(37.6818394494684,16.8896155542583,-1.58749686283055));
#169573=CARTESIAN_POINT('Ctrl Pts',(37.6808837790525,16.8776854655275,-1.85092857687063));
#169574=CARTESIAN_POINT('Ctrl Pts',(37.6796919347013,16.8627475693438,-2.11496323925901));
#169575=CARTESIAN_POINT('Ctrl Pts',(37.6782421309094,16.8447692658226,-2.37953011096301));
#169576=CARTESIAN_POINT('Ctrl Pts',(37.6771265421743,16.830935398788,-2.58310788016746));
#169577=CARTESIAN_POINT('Ctrl Pts',(37.6758586480912,16.8152949680196,-2.78706461269959));
#169578=CARTESIAN_POINT('Ctrl Pts',(37.6744464866802,16.7978338566875,-2.99120437122007));
#169579=CARTESIAN_POINT('Ctrl Pts',(37.6740321976202,16.7927112500622,-3.05109332442538));
#169580=CARTESIAN_POINT('Ctrl Pts',(37.6736089163171,16.7874561308731,-3.11071494281208));
#169581=CARTESIAN_POINT('Ctrl Pts',(37.6731765922391,16.7820679881559,-3.17011356001915));
#169582=CARTESIAN_POINT('Ctrl Pts',(37.6719959997406,16.7673540242656,-3.33231956579711));
#169583=CARTESIAN_POINT('Ctrl Pts',(37.6707455666381,16.7516609616766,-3.492804686427));
#169584=CARTESIAN_POINT('Ctrl Pts',(37.6694136223789,16.7349416760638,-3.65254969798757));
#169585=CARTESIAN_POINT('Ctrl Pts',(37.6685601749132,16.7242287413159,-3.75490681567617));
#169586=CARTESIAN_POINT('Ctrl Pts',(37.6676731846034,16.7130934292427,-3.85695982795663));
#169587=CARTESIAN_POINT('Ctrl Pts',(37.6667487152684,16.7015122921313,-3.95896503998955));
#169588=CARTESIAN_POINT('Ctrl Pts',(37.665306642091,16.6834469582562,-4.11808224883185));
#169589=CARTESIAN_POINT('Ctrl Pts',(37.6637742446663,16.6642921097485,-4.27712657394183));
#169590=CARTESIAN_POINT('Ctrl Pts',(37.6621403719767,16.6439201569281,-4.43697154140125));
#169591=CARTESIAN_POINT('Ctrl Pts',(37.6610901895404,16.6308259500296,-4.53971294739439));
#169592=CARTESIAN_POINT('Ctrl Pts',(37.6599980009714,16.6172278877262,-4.64278508072804));
#169593=CARTESIAN_POINT('Ctrl Pts',(37.6588600171528,16.6030808298185,-4.74641838392531));
#169594=CARTESIAN_POINT('Ctrl Pts',(37.657119320718,16.5814410377048,-4.90493919806702));
#169595=CARTESIAN_POINT('Ctrl Pts',(37.6552680517578,16.5585216278763,-5.06477985982275));
#169596=CARTESIAN_POINT('Ctrl Pts',(37.6532832560602,16.5341212991504,-5.22679404690265));
#169597=CARTESIAN_POINT('Ctrl Pts',(37.6520476529005,16.5189312605446,-5.32765341581011));
#169598=CARTESIAN_POINT('Ctrl Pts',(37.6507602197946,16.5031663188093,-5.42935499142178));
#169599=CARTESIAN_POINT('Ctrl Pts',(37.6494145427316,16.4867678402838,-5.5321030305694));
#169600=CARTESIAN_POINT('Ctrl Pts',(37.6477264810273,16.4661970478038,-5.66099356073221));
#169601=CARTESIAN_POINT('Ctrl Pts',(37.6459475667309,16.4446329529361,-5.79151094819494));
#169602=CARTESIAN_POINT('Ctrl Pts',(37.644066757918,16.4219341838855,-5.92408495149976));
#169603=CARTESIAN_POINT('Ctrl Pts',(37.6438356927928,16.4191455464254,-5.94037221496444));
#169604=CARTESIAN_POINT('Ctrl Pts',(37.6436030908199,16.4163397511713,-5.95669052135907));
#169605=CARTESIAN_POINT('Ctrl Pts',(37.6433689332556,16.4135165092223,-5.97304067012239));
#169606=CARTESIAN_POINT('Ctrl Pts',(37.6432522096014,16.4121091700319,-5.98119094754805));
#169607=CARTESIAN_POINT('Ctrl Pts',(37.6431350999015,16.410697496005,-5.98934913810345));
#169608=CARTESIAN_POINT('Ctrl Pts',(37.6430176009401,16.4092814491186,-5.99751533932816));
#169609=CARTESIAN_POINT('Ctrl Pts',(37.6430052115928,16.4091321380398,-5.99837640143482));
#169610=CARTESIAN_POINT('Ctrl Pts',(37.6429935354935,16.4089890431194,-5.9992013678156));
#169611=CARTESIAN_POINT('Ctrl Pts',(37.6429823705982,16.4088504836746,-6.00000000745612));
#169612=CARTESIAN_POINT('Ctrl Pts',(12.322789768,18.544964634,-6.));
#169613=CARTESIAN_POINT('Ctrl Pts',(20.805042813,18.10080432,-6.));
#169614=CARTESIAN_POINT('Ctrl Pts',(29.218799064,17.39099662,-6.));
#169615=CARTESIAN_POINT('Ctrl Pts',(37.696982896,16.402554748,-6.));
#169616=CARTESIAN_POINT('Ctrl Pts',(37.745830911,16.396859728,-6.));
#169617=CARTESIAN_POINT('Ctrl Pts',(37.794678925,16.391164709,-6.));
#169618=CARTESIAN_POINT('Ctrl Pts',(12.327415095,18.633221115,-5.492095716));
#169619=CARTESIAN_POINT('Ctrl Pts',(20.811370844,18.187540467,-5.499959461));
#169620=CARTESIAN_POINT('Ctrl Pts',(29.226829801,17.476212432,-5.507823206));
#169621=CARTESIAN_POINT('Ctrl Pts',(37.706726206,16.486241416,-5.515732521));
#169622=CARTESIAN_POINT('Ctrl Pts',(37.755584088,16.480537586,-5.515778092));
#169623=CARTESIAN_POINT('Ctrl Pts',(37.80444197,16.474833756,-5.515823662));
#169624=CARTESIAN_POINT('Ctrl Pts',(12.33537271,18.785061463,-4.485838856));
#169625=CARTESIAN_POINT('Ctrl Pts',(20.822453735,18.33838052,-4.501664827));
#169626=CARTESIAN_POINT('Ctrl Pts',(29.241037967,17.626052192,-4.517490798));
#169627=CARTESIAN_POINT('Ctrl Pts',(37.724077758,16.635075084,-4.53340848));
#169628=CARTESIAN_POINT('Ctrl Pts',(37.772953751,16.629365458,-4.533500192));
#169629=CARTESIAN_POINT('Ctrl Pts',(37.821829744,16.623655831,-4.533591903));
#169630=CARTESIAN_POINT('Ctrl Pts',(12.343761894,18.945136627,-2.991664426));
#169631=CARTESIAN_POINT('Ctrl Pts',(20.83436062,18.49923972,-3.004604703));
#169632=CARTESIAN_POINT('Ctrl Pts',(29.256462552,17.787695426,-3.01754498));
#169633=CARTESIAN_POINT('Ctrl Pts',(37.743040429,16.797506898,-3.030560246));
#169634=CARTESIAN_POINT('Ctrl Pts',(37.791936807,16.791801815,-3.030635235));
#169635=CARTESIAN_POINT('Ctrl Pts',(37.840833185,16.786096731,-3.030710224));
#169636=CARTESIAN_POINT('Ctrl Pts',(12.348776536,19.0408217,-1.50111232));
#169637=CARTESIAN_POINT('Ctrl Pts',(20.841516732,18.59571313,-1.505109267));
#169638=CARTESIAN_POINT('Ctrl Pts',(29.265760136,17.884957174,-1.509106213));
#169639=CARTESIAN_POINT('Ctrl Pts',(37.754491893,16.895561551,-1.513126323));
#169640=CARTESIAN_POINT('Ctrl Pts',(37.803400681,16.889861036,-1.513149485));
#169641=CARTESIAN_POINT('Ctrl Pts',(37.852309468,16.884160521,-1.513172647));
#169642=CARTESIAN_POINT('Ctrl Pts',(12.349906111,19.062375268,-0.502481944));
#169643=CARTESIAN_POINT('Ctrl Pts',(20.843107004,18.617265471,-0.502481944));
#169644=CARTESIAN_POINT('Ctrl Pts',(29.267811104,17.906508286,-0.502481944));
#169645=CARTESIAN_POINT('Ctrl Pts',(37.757006229,16.917111428,-0.502481944));
#169646=CARTESIAN_POINT('Ctrl Pts',(37.805917686,16.911410906,-0.502481944));
#169647=CARTESIAN_POINT('Ctrl Pts',(37.854829143,16.905710385,-0.502481944));
#169648=CARTESIAN_POINT('Ctrl Pts',(12.349906111,19.062375268,0.502481944));
#169649=CARTESIAN_POINT('Ctrl Pts',(20.843107004,18.617265471,0.502481944));
#169650=CARTESIAN_POINT('Ctrl Pts',(29.267811104,17.906508286,0.502481944));
#169651=CARTESIAN_POINT('Ctrl Pts',(37.757006229,16.917111428,0.502481944));
#169652=CARTESIAN_POINT('Ctrl Pts',(37.805917686,16.911410906,0.502481944));
#169653=CARTESIAN_POINT('Ctrl Pts',(37.854829143,16.905710385,0.502481944));
#169654=CARTESIAN_POINT('Ctrl Pts',(12.348776556,19.040822084,1.501116545));
#169655=CARTESIAN_POINT('Ctrl Pts',(20.841516748,18.595713412,1.505111951));
#169656=CARTESIAN_POINT('Ctrl Pts',(29.265760148,17.884957354,1.509107358));
#169657=CARTESIAN_POINT('Ctrl Pts',(37.754491901,16.895561629,1.513125918));
#169658=CARTESIAN_POINT('Ctrl Pts',(37.803400688,16.889861114,1.513149071));
#169659=CARTESIAN_POINT('Ctrl Pts',(37.852309476,16.884160598,1.513172225));
#169660=CARTESIAN_POINT('Ctrl Pts',(12.343761876,18.945136279,2.991660231));
#169661=CARTESIAN_POINT('Ctrl Pts',(20.834360626,18.499239639,3.004600343));
#169662=CARTESIAN_POINT('Ctrl Pts',(29.256462584,17.787695613,3.017540455));
#169663=CARTESIAN_POINT('Ctrl Pts',(37.743040486,16.797507354,3.030555555));
#169664=CARTESIAN_POINT('Ctrl Pts',(37.791936864,16.791802272,3.030630543));
#169665=CARTESIAN_POINT('Ctrl Pts',(37.840833242,16.786097191,3.030705531));
#169666=CARTESIAN_POINT('Ctrl Pts',(12.335372745,18.785062123,4.485837733));
#169667=CARTESIAN_POINT('Ctrl Pts',(20.822453727,18.338380717,4.501665456));
#169668=CARTESIAN_POINT('Ctrl Pts',(29.241037917,17.626051924,4.517493179));
#169669=CARTESIAN_POINT('Ctrl Pts',(37.724077666,16.63507435,4.533412624));
#169670=CARTESIAN_POINT('Ctrl Pts',(37.772953659,16.629364721,4.533504345));
#169671=CARTESIAN_POINT('Ctrl Pts',(37.821829651,16.623655091,4.533596067));
#169672=CARTESIAN_POINT('Ctrl Pts',(12.327415095,18.633221115,5.492095716));
#169673=CARTESIAN_POINT('Ctrl Pts',(20.811370844,18.187540467,5.499959461));
#169674=CARTESIAN_POINT('Ctrl Pts',(29.226829801,17.476212432,5.507823206));
#169675=CARTESIAN_POINT('Ctrl Pts',(37.706726206,16.486241416,5.515732521));
#169676=CARTESIAN_POINT('Ctrl Pts',(37.755584088,16.480537586,5.515778092));
#169677=CARTESIAN_POINT('Ctrl Pts',(37.80444197,16.474833756,5.515823662));
#169678=CARTESIAN_POINT('Ctrl Pts',(12.322789768,18.544964634,6.));
#169679=CARTESIAN_POINT('Ctrl Pts',(20.805042813,18.10080432,6.));
#169680=CARTESIAN_POINT('Ctrl Pts',(29.218799064,17.39099662,6.));
#169681=CARTESIAN_POINT('Ctrl Pts',(37.696982896,16.402554748,6.));
#169682=CARTESIAN_POINT('Ctrl Pts',(37.745830911,16.396859728,6.));
#169683=CARTESIAN_POINT('Ctrl Pts',(37.794678925,16.391164709,6.));
#169684=CARTESIAN_POINT('',(12.3227897708766,18.5449646343773,-6.00000000073637));
#169685=CARTESIAN_POINT('Ctrl Pts',(37.6429823592795,16.4088504483972,-6.));
#169686=CARTESIAN_POINT('Ctrl Pts',(29.215370394797,17.3912858606986,-6.));
#169687=CARTESIAN_POINT('Ctrl Pts',(20.8033145247598,18.1008948191318,-6.));
#169688=CARTESIAN_POINT('Ctrl Pts',(12.322789770849,18.5449646338508,-6.));
#169689=CARTESIAN_POINT('',(12.3227897695898,18.5449646340518,5.99999999988931));
#169690=CARTESIAN_POINT('Origin',(10.5181481816952,-15.8896585700102,-1.0547118733939E-13));
#169691=CARTESIAN_POINT('Ctrl Pts',(37.6429822858137,16.4088504569613,6.));
#169692=CARTESIAN_POINT('Ctrl Pts',(29.2153703459101,17.3912858648225,6.));
#169693=CARTESIAN_POINT('Ctrl Pts',(20.8033145001175,18.1008948204222,6.));
#169694=CARTESIAN_POINT('Ctrl Pts',(12.322789770849,18.5449646338508,6.));
#169695=CARTESIAN_POINT('Ctrl Pts',(5.858730877,11.405676811,-6.07136287));
#169696=CARTESIAN_POINT('Ctrl Pts',(6.548706819,14.528840635,-6.62786704299999));
#169697=CARTESIAN_POINT('Ctrl Pts',(9.792928396,14.486011331,-6.742357133));
#169698=CARTESIAN_POINT('Ctrl Pts',(5.861554445,11.418457643,-5.945982486));
#169699=CARTESIAN_POINT('Ctrl Pts',(6.545583205,14.547062662,-6.502968281));
#169700=CARTESIAN_POINT('Ctrl Pts',(9.793925217,14.507341164,-6.616966439));
#169701=CARTESIAN_POINT('Ctrl Pts',(5.864335028,11.43124245,-5.820600981));
#169702=CARTESIAN_POINT('Ctrl Pts',(6.542390433,14.565263133,-6.378128918));
#169703=CARTESIAN_POINT('Ctrl Pts',(9.794847306,14.528672929,-6.491571576));
#169704=CARTESIAN_POINT('Ctrl Pts',(5.868441471,11.450425087,-5.632526913));
#169705=CARTESIAN_POINT('Ctrl Pts',(6.537496645,14.592536166,-6.190912081));
#169706=CARTESIAN_POINT('Ctrl Pts',(9.796116904,14.560672554,-6.303472858));
#169707=CARTESIAN_POINT('Ctrl Pts',(5.869799547,11.456820204,-5.569835256));
#169708=CARTESIAN_POINT('Ctrl Pts',(6.535847312,14.601625942,-6.128490283));
#169709=CARTESIAN_POINT('Ctrl Pts',(9.79652118,14.571339425,-6.240772214));
#169710=CARTESIAN_POINT('Ctrl Pts',(5.871820559,11.466414169,-5.475797302));
#169711=CARTESIAN_POINT('Ctrl Pts',(6.53334715300001,14.615253408,-6.03486809500001));
#169712=CARTESIAN_POINT('Ctrl Pts',(9.79709903,14.58734011,-6.14671962));
#169713=CARTESIAN_POINT('Ctrl Pts',(5.872491546,11.469612372,-5.44445124));
#169714=CARTESIAN_POINT('Ctrl Pts',(6.53250924799999,14.619795542,-6.003656642));
#169715=CARTESIAN_POINT('Ctrl Pts',(9.797286886,14.592673734,-6.115368484));
#169716=CARTESIAN_POINT('Ctrl Pts',(5.873494003,11.474409991,-5.397432027));
#169717=CARTESIAN_POINT('Ctrl Pts',(6.531245852,14.626606909,-5.95684208399999));
#169718=CARTESIAN_POINT('Ctrl Pts',(9.797561506,14.600674251,-6.068341371));
#169719=CARTESIAN_POINT('Ctrl Pts',(5.873827484,11.47600925,-5.381758936));
#169720=CARTESIAN_POINT('Ctrl Pts',(6.530823591,14.628877271,-5.94123621600001));
#169721=CARTESIAN_POINT('Ctrl Pts',(9.797651851,14.603341103,-6.052665598));
#169722=CARTESIAN_POINT('Ctrl Pts',(5.8743267,11.478408216,-5.35824927));
#169723=CARTESIAN_POINT('Ctrl Pts',(6.530188563,14.632282349,-5.917828068));
#169724=CARTESIAN_POINT('Ctrl Pts',(9.797785576,14.607341399,-6.029151836));
#169725=CARTESIAN_POINT('Ctrl Pts',(5.874492938,11.479207884,-5.35041271));
#169726=CARTESIAN_POINT('Ctrl Pts',(6.52997660500001,14.633417351,-5.91002509800001));
#169727=CARTESIAN_POINT('Ctrl Pts',(9.797829852,14.608674834,-6.021313898));
#169728=CARTESIAN_POINT('Ctrl Pts',(5.874742043,11.480407405,-5.338657861));
#169729=CARTESIAN_POINT('Ctrl Pts',(6.529658259,14.635119738,-5.898320807));
#169730=CARTESIAN_POINT('Ctrl Pts',(9.797895818,14.610674991,-6.009556966));
#169731=CARTESIAN_POINT('Ctrl Pts',(5.874825036,11.480807249,-5.334739577));
#169732=CARTESIAN_POINT('Ctrl Pts',(6.529552073,14.635687194,-5.894419313));
#169733=CARTESIAN_POINT('Ctrl Pts',(9.797917731,14.611341711,-6.005637984));
#169734=CARTESIAN_POINT('Ctrl Pts',(5.874990938,11.481606943,-5.326903007));
#169735=CARTESIAN_POINT('Ctrl Pts',(6.529339564,14.636822076,-5.886616319));
#169736=CARTESIAN_POINT('Ctrl Pts',(9.797961409,14.612675152,-5.997800012));
#169737=CARTESIAN_POINT('Ctrl Pts',(5.875073803,11.48200658,-5.322984668));
#169738=CARTESIAN_POINT('Ctrl Pts',(6.529247215,14.637456319,-5.882064614));
#169739=CARTESIAN_POINT('Ctrl Pts',(9.797957984,14.613472876,-5.993108854));
#169740=CARTESIAN_POINT('Ctrl Pts',(5.880449993,11.50794786,-5.068283718));
#169741=CARTESIAN_POINT('Ctrl Pts',(6.52291790199999,14.677089485,-5.601170537));
#169742=CARTESIAN_POINT('Ctrl Pts',(9.79831837,14.662187405,-5.706218389));
#169743=CARTESIAN_POINT('Ctrl Pts',(5.885197279,11.531688249,-4.817044188));
#169744=CARTESIAN_POINT('Ctrl Pts',(6.51682845,14.71329959,-5.32418104));
#169745=CARTESIAN_POINT('Ctrl Pts',(9.798332145,14.70673276,-5.423259124));
#169746=CARTESIAN_POINT('Ctrl Pts',(5.898005992,11.597492508,-4.061961581));
#169747=CARTESIAN_POINT('Ctrl Pts',(6.49931662200001,14.813695466,-4.490653682));
#169748=CARTESIAN_POINT('Ctrl Pts',(9.797716555,14.830132736,-4.572917229));
#169749=CARTESIAN_POINT('Ctrl Pts',(5.904645385,11.634142573,-3.556755763));
#169750=CARTESIAN_POINT('Ctrl Pts',(6.488702427,14.869437222,-3.933025041));
#169751=CARTESIAN_POINT('Ctrl Pts',(9.796448164,14.89875956,-4.004074322));
#169752=CARTESIAN_POINT('Ctrl Pts',(5.912372151,11.678198728,-2.796229212));
#169753=CARTESIAN_POINT('Ctrl Pts',(6.475482211,14.936409695,-3.092941977));
#169754=CARTESIAN_POINT('Ctrl Pts',(9.794420092,14.981209295,-3.147746793));
#169755=CARTESIAN_POINT('Ctrl Pts',(5.91457177,11.691057231,-2.542330331));
#169756=CARTESIAN_POINT('Ctrl Pts',(6.471523067,14.955948086,-2.812266956));
#169757=CARTESIAN_POINT('Ctrl Pts',(9.793718352,15.005264335,-2.861852142));
#169758=CARTESIAN_POINT('Ctrl Pts',(5.918286894,11.713083094,-2.034565643));
#169759=CARTESIAN_POINT('Ctrl Pts',(6.464643913,14.98940459,-2.250799451));
#169760=CARTESIAN_POINT('Ctrl Pts',(9.792409909,15.046453364,-2.290188755));
#169761=CARTESIAN_POINT('Ctrl Pts',(5.919803707,11.722258,-1.780587582));
#169762=CARTESIAN_POINT('Ctrl Pts',(6.461723305,15.00332776,-1.969936019));
#169763=CARTESIAN_POINT('Ctrl Pts',(9.791803155,15.063602815,-2.004281364));
#169764=CARTESIAN_POINT('Ctrl Pts',(5.923413308,11.744282385,-1.01836763));
#169765=CARTESIAN_POINT('Ctrl Pts',(6.454651993,15.036755268,-1.126615399));
#169766=CARTESIAN_POINT('Ctrl Pts',(9.790282759,15.104762632,-1.146284737));
#169767=CARTESIAN_POINT('Ctrl Pts',(5.924576429,11.751636075,-0.509840295));
#169768=CARTESIAN_POINT('Ctrl Pts',(6.452217343,15.04789064,-0.564196861));
#169769=CARTESIAN_POINT('Ctrl Pts',(9.789690097,15.118496245,-0.573921954));
#169770=CARTESIAN_POINT('Ctrl Pts',(5.924578584,11.751649539,0.253521895));
#169771=CARTESIAN_POINT('Ctrl Pts',(6.452212928,15.047911057,0.280551221));
#169772=CARTESIAN_POINT('Ctrl Pts',(9.789689064,15.118521399,0.285386979));
#169773=CARTESIAN_POINT('Ctrl Pts',(5.924286082,11.749816719,0.508071237));
#169774=CARTESIAN_POINT('Ctrl Pts',(6.452815375,15.045132787,0.562189979));
#169775=CARTESIAN_POINT('Ctrl Pts',(9.789831464,15.115097648,0.571910231));
#169776=CARTESIAN_POINT('Ctrl Pts',(5.923102816,11.742468341,1.017360989));
#169777=CARTESIAN_POINT('Ctrl Pts',(6.45521236800001,15.033988844,1.125683846));
#169778=CARTESIAN_POINT('Ctrl Pts',(9.790381318,15.101369381,1.145167357));
#169779=CARTESIAN_POINT('Ctrl Pts',(5.922211942,11.736952169,1.272010148));
#169780=CARTESIAN_POINT('Ctrl Pts',(6.457006545,15.025624748,1.407373847));
#169781=CARTESIAN_POINT('Ctrl Pts',(9.790788763,15.091063707,1.431798692));
#169782=CARTESIAN_POINT('Ctrl Pts',(5.918600378,11.714915645,2.03477498));
#169783=CARTESIAN_POINT('Ctrl Pts',(6.464078579,14.992194076,2.250912567));
#169784=CARTESIAN_POINT('Ctrl Pts',(9.792310053,15.04988121,2.290408636));
#169785=CARTESIAN_POINT('Ctrl Pts',(5.914950781,11.692903678,2.542161979));
#169786=CARTESIAN_POINT('Ctrl Pts',(6.47106091500001,14.958803958,2.811788959));
#169787=CARTESIAN_POINT('Ctrl Pts',(9.793742403,15.008729087,2.861675555));
#169788=CARTESIAN_POINT('Ctrl Pts',(5.904669074,11.634275422,3.5546825));
#169789=CARTESIAN_POINT('Ctrl Pts',(6.488663272,14.869639199,3.930736359));
#169790=CARTESIAN_POINT('Ctrl Pts',(9.796442812,14.899008251,4.001739907));
#169791=CARTESIAN_POINT('Ctrl Pts',(5.898038406,11.597664362,4.059816839));
#169792=CARTESIAN_POINT('Ctrl Pts',(6.499269057,14.813957462,4.48828503));
#169793=CARTESIAN_POINT('Ctrl Pts',(9.797713013,14.830454794,4.570502105));
#169794=CARTESIAN_POINT('Ctrl Pts',(5.885220146,11.531803076,4.815812574));
#169795=CARTESIAN_POINT('Ctrl Pts',(6.51679881700001,14.713474789,5.322822554));
#169796=CARTESIAN_POINT('Ctrl Pts',(9.798332034,14.706948197,5.421872036));
#169797=CARTESIAN_POINT('Ctrl Pts',(5.880467048,11.508031537,5.067432231));
#169798=CARTESIAN_POINT('Ctrl Pts',(6.52289699300001,14.677217237,5.600231576));
#169799=CARTESIAN_POINT('Ctrl Pts',(9.798319009,14.66234448,5.705259343));
#169800=CARTESIAN_POINT('Ctrl Pts',(5.875128186,11.482268981,5.320408522));
#169801=CARTESIAN_POINT('Ctrl Pts',(6.52918324499999,14.637856905,5.87922574199999));
#169802=CARTESIAN_POINT('Ctrl Pts',(9.797961633,14.613965632,5.990207131));
#169803=CARTESIAN_POINT('Ctrl Pts',(5.875086766,11.482069161,5.322369546));
#169804=CARTESIAN_POINT('Ctrl Pts',(6.529231947,14.637551851,5.88138678300001));
#169805=CARTESIAN_POINT('Ctrl Pts',(9.797958842,14.613590394,5.992415993));
#169806=CARTESIAN_POINT('Ctrl Pts',(5.87500386,11.481669303,5.326291527));
#169807=CARTESIAN_POINT('Ctrl Pts',(6.52932936600001,14.636941405,5.88570877400001));
#169808=CARTESIAN_POINT('Ctrl Pts',(9.797953217,14.612839501,5.996833648));
#169809=CARTESIAN_POINT('Ctrl Pts',(5.874962367,11.481469234,5.328252476));
#169810=CARTESIAN_POINT('Ctrl Pts',(6.529376155,14.63662664,5.887960052));
#169811=CARTESIAN_POINT('Ctrl Pts',(9.797953883,14.612445531,5.999149722));
#169812=CARTESIAN_POINT('Ctrl Pts',(5.874837833,11.480868914,5.334135288));
#169813=CARTESIAN_POINT('Ctrl Pts',(6.529535693,14.635774708,5.893817613));
#169814=CARTESIAN_POINT('Ctrl Pts',(9.797921106,14.611444534,6.005033587));
#169815=CARTESIAN_POINT('Ctrl Pts',(5.874754768,11.480468704,5.338057161));
#169816=CARTESIAN_POINT('Ctrl Pts',(6.529641983,14.635206734,5.89772268099999));
#169817=CARTESIAN_POINT('Ctrl Pts',(9.79789918,14.610777204,6.008956159));
#169818=CARTESIAN_POINT('Ctrl Pts',(5.874505448,11.479268083,5.349822774));
#169819=CARTESIAN_POINT('Ctrl Pts',(6.529960642,14.633502793,5.909437691));
#169820=CARTESIAN_POINT('Ctrl Pts',(9.797833178,14.608775215,6.020723859));
#169821=CARTESIAN_POINT('Ctrl Pts',(5.874339066,11.478467682,5.357666509));
#169822=CARTESIAN_POINT('Ctrl Pts',(6.530172808,14.632366755,5.917247805));
#169823=CARTESIAN_POINT('Ctrl Pts',(9.797788876,14.607440559,6.028568973));
#169824=CARTESIAN_POINT('Ctrl Pts',(5.873839418,11.476066519,5.381197693));
#169825=CARTESIAN_POINT('Ctrl Pts',(6.53080845700001,14.628958568,5.940677378));
#169826=CARTESIAN_POINT('Ctrl Pts',(9.797655073,14.603436601,6.052104258));
#169827=CARTESIAN_POINT('Ctrl Pts',(5.873505647,11.474465796,5.39688512));
#169828=CARTESIAN_POINT('Ctrl Pts',(6.531231131,14.626686136,5.956297521));
#169829=CARTESIAN_POINT('Ctrl Pts',(9.797564672,14.600767309,6.067794371));
#169830=CARTESIAN_POINT('Ctrl Pts',(5.87250232,11.469663788,5.443947316));
#169831=CARTESIAN_POINT('Ctrl Pts',(6.532495757,14.619868559,6.003154875));
#169832=CARTESIAN_POINT('Ctrl Pts',(9.797289883,14.592759478,6.114864478));
#169833=CARTESIAN_POINT('Ctrl Pts',(5.871830748,11.466462662,5.475322));
#169834=CARTESIAN_POINT('Ctrl Pts',(6.533334472,14.615322287,6.03439482699999));
#169835=CARTESIAN_POINT('Ctrl Pts',(9.797101905,14.587420984,6.146244242));
#169836=CARTESIAN_POINT('Ctrl Pts',(5.869807969,11.456859941,5.569445715));
#169837=CARTESIAN_POINT('Ctrl Pts',(6.535837037,14.601682421,6.128102391));
#169838=CARTESIAN_POINT('Ctrl Pts',(9.796523664,14.571405705,6.240382616));
#169839=CARTESIAN_POINT('Ctrl Pts',(5.868448699,11.450459003,5.632194411));
#169840=CARTESIAN_POINT('Ctrl Pts',(6.53748793900001,14.592584389,6.190580983));
#169841=CARTESIAN_POINT('Ctrl Pts',(9.796119093,14.560729128,6.30314031));
#169842=CARTESIAN_POINT('Ctrl Pts',(5.864338623,11.431258947,5.820439191));
#169843=CARTESIAN_POINT('Ctrl Pts',(6.542386322,14.565286638,6.377967716));
#169844=CARTESIAN_POINT('Ctrl Pts',(9.794848509,14.528700455,6.49140977));
#169845=CARTESIAN_POINT('Ctrl Pts',(5.861555552,11.418462588,5.945933968));
#169846=CARTESIAN_POINT('Ctrl Pts',(6.545582018,14.54706973,6.502919861));
#169847=CARTESIAN_POINT('Ctrl Pts',(9.793925628,14.507349417,6.616917918));
#169848=CARTESIAN_POINT('Ctrl Pts',(5.85872943,11.405670264,6.071427099));
#169849=CARTESIAN_POINT('Ctrl Pts',(6.54870841900001,14.528831305,6.627930994));
#169850=CARTESIAN_POINT('Ctrl Pts',(9.792927885,14.486000404,6.742421368));
#169851=CARTESIAN_POINT('Ctrl Pts',(5.86033332555925,11.4129517033987,-6.));
#169852=CARTESIAN_POINT('Ctrl Pts',(5.95551424490732,11.8463401914417,-6.));
#169853=CARTESIAN_POINT('Ctrl Pts',(6.12009715916116,12.2617765317534,-5.99999999999951));
#169854=CARTESIAN_POINT('Ctrl Pts',(6.59014416096763,13.0477845608693,-5.99999999999951));
#169855=CARTESIAN_POINT('Ctrl Pts',(6.90068104724246,13.4082770775861,-6.));
#169856=CARTESIAN_POINT('Ctrl Pts',(7.63159956820147,14.0058478634451,-6.));
#169857=CARTESIAN_POINT('Ctrl Pts',(8.04643932506048,14.2383905687456,-6.00000000000029));
#169858=CARTESIAN_POINT('Ctrl Pts',(8.91231545030028,14.5386899633179,-6.00000000000029));
#169859=CARTESIAN_POINT('Ctrl Pts',(9.35349561644513,14.6130197564008,-6.));
#169860=CARTESIAN_POINT('Ctrl Pts',(9.7979474647987,14.6123008532225,-6.));
#169861=CARTESIAN_POINT('Ctrl Pts',(5.86033332508859,11.4129517037665,6.));
#169862=CARTESIAN_POINT('Ctrl Pts',(5.95551427440473,11.8463403275766,6.));
#169863=CARTESIAN_POINT('Ctrl Pts',(6.12009726163233,12.2617767913913,5.99999999999943));
#169864=CARTESIAN_POINT('Ctrl Pts',(6.59014435623358,13.0477847950603,5.99999999999943));
#169865=CARTESIAN_POINT('Ctrl Pts',(6.90068118868703,13.4082772046647,5.99999999999999));
#169866=CARTESIAN_POINT('Ctrl Pts',(7.63160004128257,14.005848238828,5.99999999999999));
#169867=CARTESIAN_POINT('Ctrl Pts',(8.0464403159652,14.2383911178095,6.00000000000091));
#169868=CARTESIAN_POINT('Ctrl Pts',(8.91231692039178,14.5386902793529,6.00000000000091));
#169869=CARTESIAN_POINT('Ctrl Pts',(9.35349612030971,14.6130195934359,6.));
#169870=CARTESIAN_POINT('Ctrl Pts',(9.79794788833258,14.6123008700064,6.));
#169871=CARTESIAN_POINT('Origin',(3.229571164,9.085011286,3.));
#169872=CARTESIAN_POINT('',(3.23862872955019,9.08469498921557,-3.));
#169873=CARTESIAN_POINT('',(3.23862872928097,9.08469498922496,3.));
#169874=CARTESIAN_POINT('Origin',(-0.113430008273151,9.20175145934795,-6.50521302475128E-16));
#169875=CARTESIAN_POINT('',(3.229571164,9.085011286,-3.));
#169876=CARTESIAN_POINT('',(3.229571164,9.085011286,3.));
#169877=CARTESIAN_POINT('Origin',(-6.375213959,6.951087372,3.));
#169878=CARTESIAN_POINT('',(3.58379069455313,18.9688404665487,3.00000000023314));
#169879=CARTESIAN_POINT('Origin',(21.843846343214,-25.3175681408131,2.99694995567449));
#169880=CARTESIAN_POINT('',(3.58379069437062,18.968840466356,3.));
#169881=CARTESIAN_POINT('Origin',(-6.59507738,6.962404107,6.));
#169882=CARTESIAN_POINT('Ctrl Pts',(0.0871991419853988,18.6993663253053,
6.));
#169883=CARTESIAN_POINT('Ctrl Pts',(4.15193489758751,18.8818690260965,6.));
#169884=CARTESIAN_POINT('Ctrl Pts',(8.24326974937625,18.7587632189196,6.));
#169885=CARTESIAN_POINT('Ctrl Pts',(12.3227897680015,18.5449646340289,5.99999999983395));
#169886=CARTESIAN_POINT('Origin',(-6.59507738,6.962404107,-6.));
#169887=CARTESIAN_POINT('Ctrl Pts',(12.3227897708861,18.5449646345585,-6.00000000157715));
#169888=CARTESIAN_POINT('Ctrl Pts',(8.24326974936394,18.7587632189203,-6.));
#169889=CARTESIAN_POINT('Ctrl Pts',(4.15193489750702,18.8818690260931,-6.));
#169890=CARTESIAN_POINT('Ctrl Pts',(0.0871991420529483,18.6993663237096,
-6.00000000357678));
#169891=CARTESIAN_POINT('Ctrl Pts',(-0.48281518308,18.67128531332,-6.12572604072));
#169892=CARTESIAN_POINT('Ctrl Pts',(3.76893576836,18.88303868432,-6.11941794432));
#169893=CARTESIAN_POINT('Ctrl Pts',(8.05180007692,18.74907244304,-6.11320540872));
#169894=CARTESIAN_POINT('Ctrl Pts',(12.32175884152,18.52529338632,-6.11320540872));
#169895=CARTESIAN_POINT('Ctrl Pts',(-0.48280968572,18.67143671988,-6.08381736048));
#169896=CARTESIAN_POINT('Ctrl Pts',(3.76905856124,18.88642015488,-6.07961196288));
#169897=CARTESIAN_POINT('Ctrl Pts',(8.05203996028,18.75563496336,-6.07547027248));
#169898=CARTESIAN_POINT('Ctrl Pts',(12.32210248368,18.53185046888,-6.07547027248));
#169899=CARTESIAN_POINT('Ctrl Pts',(-0.48280418836,18.67158812644,-6.04190868024));
#169900=CARTESIAN_POINT('Ctrl Pts',(3.76918135412,18.88980162544,-6.03980598144));
#169901=CARTESIAN_POINT('Ctrl Pts',(8.05227984364,18.76219748368,-6.03773513624));
#169902=CARTESIAN_POINT('Ctrl Pts',(12.32244612584,18.53840755144,-6.03773513624));
#169903=CARTESIAN_POINT('Ctrl Pts',(-0.482798691,18.671739533,-6.));
#169904=CARTESIAN_POINT('Ctrl Pts',(3.769304147,18.893183096,-6.));
#169905=CARTESIAN_POINT('Ctrl Pts',(8.052519727,18.768760004,-6.));
#169906=CARTESIAN_POINT('Ctrl Pts',(12.322789768,18.544964634,-6.));
#169907=CARTESIAN_POINT('Ctrl Pts',(-0.482729974,18.673632115,-5.476141497));
#169908=CARTESIAN_POINT('Ctrl Pts',(3.770839058,18.935451478,-5.502425232));
#169909=CARTESIAN_POINT('Ctrl Pts',(8.055518269,18.850791508,-5.528310797));
#169910=CARTESIAN_POINT('Ctrl Pts',(12.327085295,18.626928166,-5.528310797));
#169911=CARTESIAN_POINT('Ctrl Pts',(-0.482611485,18.677055788,-4.454466407));
#169912=CARTESIAN_POINT('Ctrl Pts',(3.773485772,19.011914848,-4.507696353));
#169913=CARTESIAN_POINT('Ctrl Pts',(8.060694204,18.999186042,-4.560119923));
#169914=CARTESIAN_POINT('Ctrl Pts',(12.334855199,18.775186756,-4.560119923));
#169915=CARTESIAN_POINT('Ctrl Pts',(-0.482499182,18.680870321,-2.963951319));
#169916=CARTESIAN_POINT('Ctrl Pts',(3.775994487,19.097107541,-3.008905852));
#169917=CARTESIAN_POINT('Ctrl Pts',(8.065619523,19.164521142,-3.053179372));
#169918=CARTESIAN_POINT('Ctrl Pts',(12.343509801,18.940326412,-3.053179372));
#169919=CARTESIAN_POINT('Ctrl Pts',(-0.482438684,18.683187901,-1.488934103));
#169920=CARTESIAN_POINT('Ctrl Pts',(3.77734606,19.148867735,-1.504611084));
#169921=CARTESIAN_POINT('Ctrl Pts',(8.068281921,19.264972886,-1.520050575));
#169922=CARTESIAN_POINT('Ctrl Pts',(12.348767127,19.040642162,-1.520050575));
#169923=CARTESIAN_POINT('Ctrl Pts',(-0.482424746,18.683689955,-0.500057262));
#169924=CARTESIAN_POINT('Ctrl Pts',(3.777657422,19.160080453,-0.501278864));
#169925=CARTESIAN_POINT('Ctrl Pts',(8.068894181,19.286733597,-0.502481975));
#169926=CARTESIAN_POINT('Ctrl Pts',(12.349906111,19.062375268,-0.502481944));
#169927=CARTESIAN_POINT('Ctrl Pts',(-0.482424746,18.683689955,0.500057262));
#169928=CARTESIAN_POINT('Ctrl Pts',(3.777657422,19.160080453,0.501278864));
#169929=CARTESIAN_POINT('Ctrl Pts',(8.068894182,19.286733597,0.502481975));
#169930=CARTESIAN_POINT('Ctrl Pts',(12.349906111,19.062375268,0.502481944));
#169931=CARTESIAN_POINT('Ctrl Pts',(-0.482438684,18.683187895,1.4889341));
#169932=CARTESIAN_POINT('Ctrl Pts',(3.777346054,19.148867586,1.50461102));
#169933=CARTESIAN_POINT('Ctrl Pts',(8.068281909,19.264972599,1.520050451));
#169934=CARTESIAN_POINT('Ctrl Pts',(12.348767112,19.040641875,1.520050451));
#169935=CARTESIAN_POINT('Ctrl Pts',(-0.482499181,18.680870356,2.96395119));
#169936=CARTESIAN_POINT('Ctrl Pts',(3.775994518,19.097108332,3.008902976));
#169937=CARTESIAN_POINT('Ctrl Pts',(8.065619583,19.164522678,3.05317379));
#169938=CARTESIAN_POINT('Ctrl Pts',(12.343509882,18.940327947,3.05317379));
#169939=CARTESIAN_POINT('Ctrl Pts',(-0.482611487,18.677055733,4.45446654));
#169940=CARTESIAN_POINT('Ctrl Pts',(3.773485724,19.011913616,4.507699318));
#169941=CARTESIAN_POINT('Ctrl Pts',(8.060694109,18.999183651,4.560125675));
#169942=CARTESIAN_POINT('Ctrl Pts',(12.334855073,18.775184367,4.560125675));
#169943=CARTESIAN_POINT('Ctrl Pts',(-0.482729974,18.673632115,5.476141497));
#169944=CARTESIAN_POINT('Ctrl Pts',(3.770839064,18.935451478,5.502425232));
#169945=CARTESIAN_POINT('Ctrl Pts',(8.055518279,18.850791507,5.528310797));
#169946=CARTESIAN_POINT('Ctrl Pts',(12.327085295,18.626928166,5.528310797));
#169947=CARTESIAN_POINT('Ctrl Pts',(-0.482798691,18.671739533,6.));
#169948=CARTESIAN_POINT('Ctrl Pts',(3.769304147,18.893183096,6.));
#169949=CARTESIAN_POINT('Ctrl Pts',(8.052519727,18.768760004,6.));
#169950=CARTESIAN_POINT('Ctrl Pts',(12.322789768,18.544964634,6.));
#169951=CARTESIAN_POINT('',(3.58379068683386,18.9688402467474,-3.00000000092337));
#169952=CARTESIAN_POINT('Origin',(21.8433741830221,-25.3164218281024,-2.99694738992876));
#169953=CARTESIAN_POINT('Ctrl Pts',(3.58379069506722,18.9688404666728,3.00000000070508));
#169954=CARTESIAN_POINT('Ctrl Pts',(3.93212928952008,19.0011909115314,2.6120451340472));
#169955=CARTESIAN_POINT('Ctrl Pts',(4.21077841803549,19.0311539303752,2.16640319802089));
#169956=CARTESIAN_POINT('Ctrl Pts',(4.62301577610162,19.0776799622152,1.14857626613188));
#169957=CARTESIAN_POINT('Ctrl Pts',(4.73453392972642,19.0915863401855,0.577867853909078));
#169958=CARTESIAN_POINT('Ctrl Pts',(4.73481426051302,19.0916201533682,-0.576113189726437));
#169959=CARTESIAN_POINT('Ctrl Pts',(4.62341089666168,19.0777265352238,-1.14728416993611));
#169960=CARTESIAN_POINT('Ctrl Pts',(4.21110962532196,19.0311893688141,-2.16587157842389));
#169961=CARTESIAN_POINT('Ctrl Pts',(3.93233425257726,19.0012095955261,-2.61181684710127));
#169962=CARTESIAN_POINT('Ctrl Pts',(3.58379068702773,18.9688402469573,-3.00000000111494));
#169963=CARTESIAN_POINT('Origin',(-0.113430008291004,9.2017514588367,-6.50521303491303E-16));
#169964=CARTESIAN_POINT('',(3.23862872920799,9.08469498834335,-3.));
#169965=CARTESIAN_POINT('Origin',(5.333796876,18.951915666,-3.));
#170238=UNCERTAINTY_MEASURE_WITH_UNIT(LENGTH_MEASURE(0.01),#170251,
'DISTANCE_ACCURACY_VALUE',
'Maximum model space distance between geometric entities at asserted c
onnectivities');
#170242=UNCERTAINTY_MEASURE_WITH_UNIT(LENGTH_MEASURE(0.01),#170251,
'DISTANCE_ACCURACY_VALUE',
'Maximum model space distance between geometric entities at asserted c
onnectivities');
#170246=(
GEOMETRIC_REPRESENTATION_CONTEXT(3)
GLOBAL_UNCERTAINTY_ASSIGNED_CONTEXT((#170238))
GLOBAL_UNIT_ASSIGNED_CONTEXT((#170251,#170253,#170254))
REPRESENTATION_CONTEXT('','3D')
);
#170250=(
GEOMETRIC_REPRESENTATION_CONTEXT(3)
GLOBAL_UNCERTAINTY_ASSIGNED_CONTEXT((#170242))
GLOBAL_UNIT_ASSIGNED_CONTEXT((#170251,#170253,#170254))
REPRESENTATION_CONTEXT('','3D')
);
#170251=(
LENGTH_UNIT()
NAMED_UNIT(*)
SI_UNIT(.MILLI.,.METRE.)
);
#170253=(
NAMED_UNIT(*)
PLANE_ANGLE_UNIT()
SI_UNIT($,.RADIAN.)
);
#170254=(
NAMED_UNIT(*)
SI_UNIT($,.STERADIAN.)
SOLID_ANGLE_UNIT()
);
#170258=SHAPE_DEFINITION_REPRESENTATION(#170265,#170278);
#170265=PRODUCT_DEFINITION_SHAPE('',$,#170286);
#170278=SHAPE_REPRESENTATION('',(#77681),#170246);
#170282=PRODUCT_DEFINITION_CONTEXT('part definition',#170305,'design');
#170286=PRODUCT_DEFINITION('2026-11-14-09-55-10-334_2','Lever arm',#170293,
#170282);
#170293=PRODUCT_DEFINITION_FORMATION('',$,#170310);
#170305=APPLICATION_CONTEXT(
'Core Data for Automotive Mechanical Design Process');
#170306=PRODUCT_CONTEXT('part definition',#170305,'mechanical');
#170310=PRODUCT('2026-11-14-09-55-10-334_2','Lever arm',$,(#170306));
#170316=PRESENTATION_STYLE_ASSIGNMENT((#170320));
#170320=SURFACE_STYLE_USAGE(.BOTH.,#170324);
#170324=SURFACE_SIDE_STYLE('',(#170328));
#170328=SURFACE_STYLE_FILL_AREA(#170332);
#170332=FILL_AREA_STYLE('Opaque(97,158,199)',(#170336));
#170336=FILL_AREA_STYLE_COLOUR('Opaque(97,158,199)',#170340);
#170340=COLOUR_RGB('Opaque(97,158,199)',0.380392156862745,0.619607843137255,
0.780392156862745);
ENDSEC;
END-ISO-10303-21;
